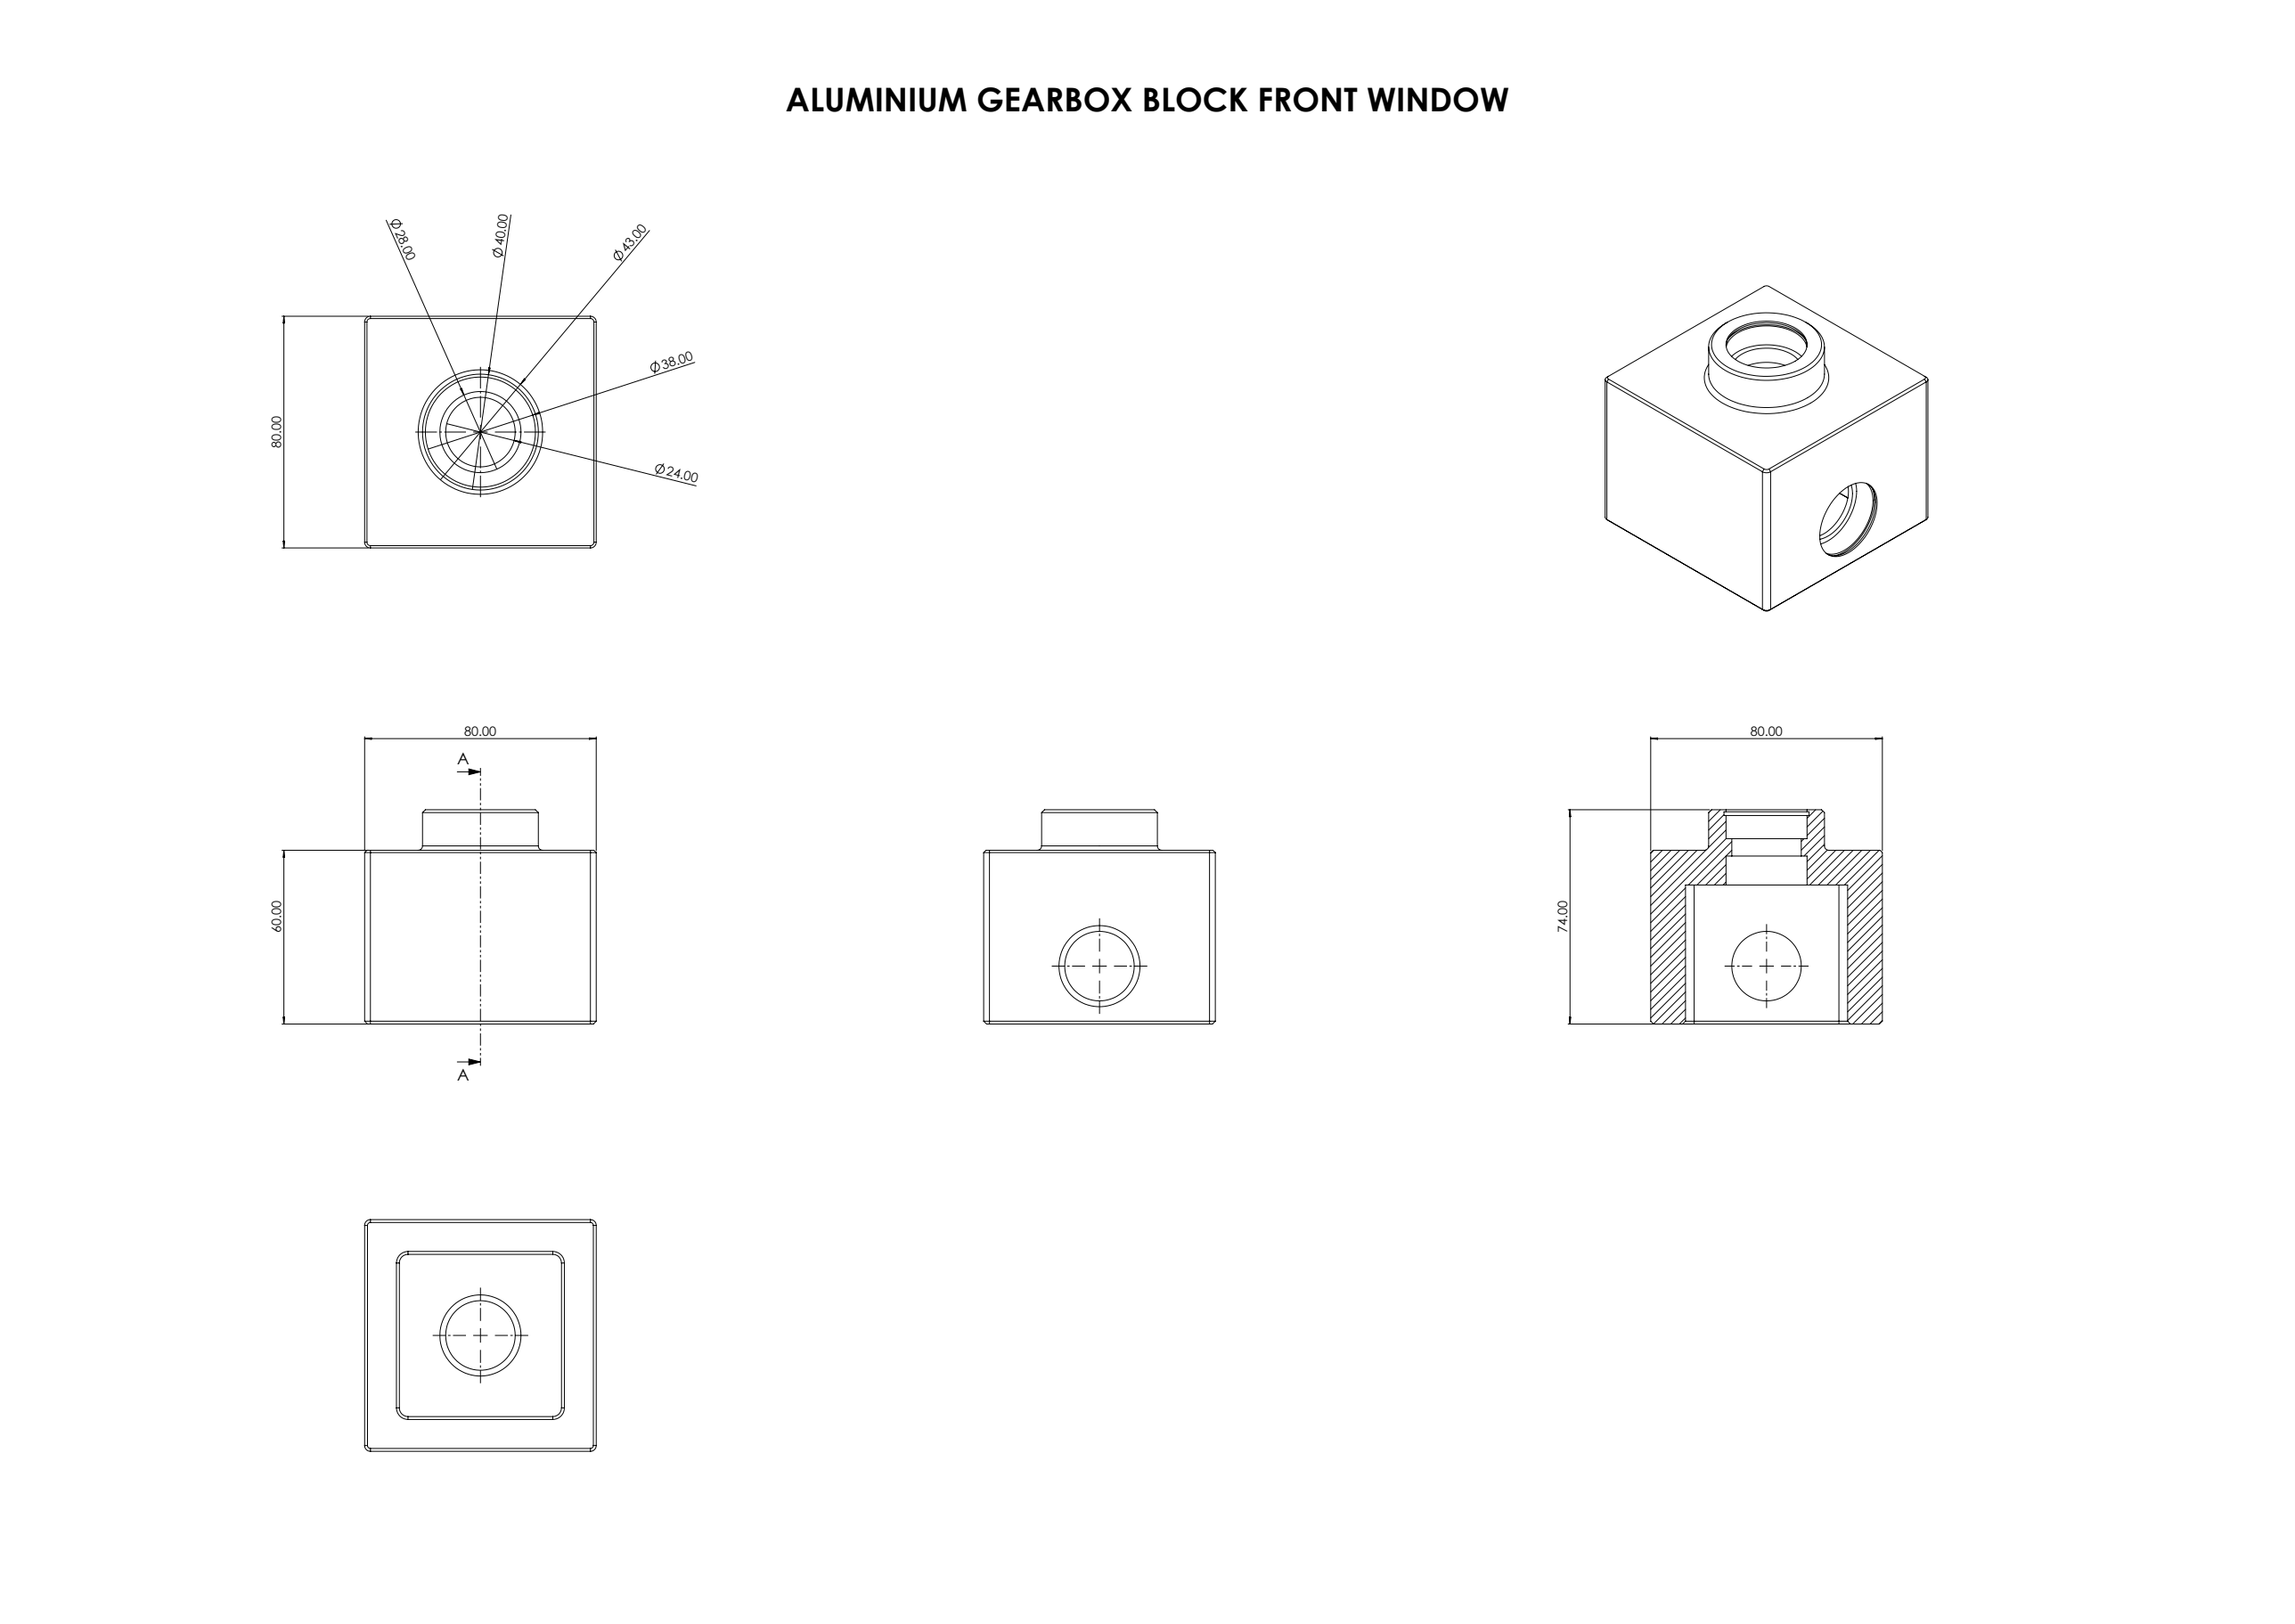
ISO-10303-21;
HEADER;
/* Generated by software containing ST-Developer
 * from STEP Tools, Inc. (www.steptools.com) 
 */

FILE_DESCRIPTION(
/* description */ (''),
/* implementation_level */ '2;1');

FILE_NAME(
/* name */ '01_Aluminium_Gearbox_Block_Front_Window.step',
/* time_stamp */ '2026-10-11T09:12:28-07:00',
/* author */ (''),
/* organization */ (''),
/* preprocessor_version */ 'ST-DEVELOPER v20.2',
/* originating_system */ 'Autodesk Translation Framework v15.15.0.0',
/* authorisation */ '');

FILE_SCHEMA (('AUTOMOTIVE_DESIGN { 1 0 10303 214 3 1 1 }'));
ENDSEC;

DATA;
#10=MECHANICAL_DESIGN_GEOMETRIC_PRESENTATION_REPRESENTATION('',(#647),#23254);
#627=SHAPE_REPRESENTATION_RELATIONSHIP('SRR','None',#23300,#637);
#637=ADVANCED_BREP_SHAPE_REPRESENTATION('',(#657),#23244);
#647=STYLED_ITEM('',(#23441),#657);
#657=MANIFOLD_SOLID_BREP('Body1',#7025);
#667=CONICAL_SURFACE('',#7210,19.5,0.785398163397451);
#668=CONICAL_SURFACE('',#7214,1.6,0.785398163397445);
#669=CONICAL_SURFACE('',#7217,1.6,0.785398163397448);
#670=CONICAL_SURFACE('',#7220,1.6,0.785398163397448);
#671=CONICAL_SURFACE('',#7223,1.6,0.785398163397445);
#672=CONICAL_SURFACE('',#7231,1.5,0.785398163397449);
#673=CONICAL_SURFACE('',#7234,1.5,0.785398163397447);
#674=CONICAL_SURFACE('',#7238,1.5,0.785398163397447);
#675=CONICAL_SURFACE('',#7242,1.5,0.785398163397449);
#676=CONICAL_SURFACE('',#7250,3.5,0.785398163397447);
#677=CONICAL_SURFACE('',#7253,3.5,0.785398163397447);
#678=CONICAL_SURFACE('',#7256,3.5,0.785398163397447);
#679=CONICAL_SURFACE('',#7259,3.5,0.785398163397447);
#759=TOROIDAL_SURFACE('',#7197,21.5,1.5);
#780=FACE_BOUND('',#1376,.T.);
#781=FACE_BOUND('',#1379,.T.);
#782=FACE_BOUND('',#1382,.T.);
#783=FACE_BOUND('',#1385,.T.);
#784=FACE_BOUND('',#1389,.T.);
#785=FACE_BOUND('',#1392,.T.);
#786=FACE_BOUND('',#1395,.T.);
#787=FACE_BOUND('',#1399,.T.);
#788=FACE_BOUND('',#1402,.T.);
#789=FACE_BOUND('',#1405,.T.);
#790=FACE_BOUND('',#1410,.T.);
#791=FACE_BOUND('',#1413,.T.);
#792=FACE_BOUND('',#1424,.T.);
#793=FACE_BOUND('',#1436,.T.);
#794=FACE_BOUND('',#1446,.T.);
#795=FACE_BOUND('',#1451,.T.);
#796=FACE_BOUND('',#1453,.T.);
#797=FACE_BOUND('',#1459,.T.);
#852=PLANE('',#7151);
#853=PLANE('',#7155);
#854=PLANE('',#7159);
#855=PLANE('',#7163);
#856=PLANE('',#7170);
#857=PLANE('',#7174);
#858=PLANE('',#7178);
#859=PLANE('',#7185);
#860=PLANE('',#7189);
#861=PLANE('',#7193);
#862=PLANE('',#7205);
#863=PLANE('',#7212);
#864=PLANE('',#7213);
#865=PLANE('',#7216);
#866=PLANE('',#7219);
#867=PLANE('',#7222);
#868=PLANE('',#7227);
#869=PLANE('',#7230);
#870=PLANE('',#7233);
#871=PLANE('',#7237);
#872=PLANE('',#7241);
#873=PLANE('',#7244);
#874=PLANE('',#7245);
#875=PLANE('',#7252);
#876=PLANE('',#7255);
#877=PLANE('',#7258);
#878=PLANE('',#7261);
#879=PLANE('',#7262);
#880=PLANE('',#7265);
#881=PLANE('',#7268);
#882=PLANE('',#7271);
#883=PLANE('',#7274);
#884=PLANE('',#7276);
#885=PLANE('',#7278);
#979=FACE_OUTER_BOUND('',#1374,.T.);
#980=FACE_OUTER_BOUND('',#1375,.T.);
#981=FACE_OUTER_BOUND('',#1377,.T.);
#982=FACE_OUTER_BOUND('',#1378,.T.);
#983=FACE_OUTER_BOUND('',#1380,.T.);
#984=FACE_OUTER_BOUND('',#1381,.T.);
#985=FACE_OUTER_BOUND('',#1383,.T.);
#986=FACE_OUTER_BOUND('',#1384,.T.);
#987=FACE_OUTER_BOUND('',#1386,.T.);
#988=FACE_OUTER_BOUND('',#1387,.T.);
#989=FACE_OUTER_BOUND('',#1388,.T.);
#990=FACE_OUTER_BOUND('',#1390,.T.);
#991=FACE_OUTER_BOUND('',#1391,.T.);
#992=FACE_OUTER_BOUND('',#1393,.T.);
#993=FACE_OUTER_BOUND('',#1394,.T.);
#994=FACE_OUTER_BOUND('',#1396,.T.);
#995=FACE_OUTER_BOUND('',#1397,.T.);
#996=FACE_OUTER_BOUND('',#1398,.T.);
#997=FACE_OUTER_BOUND('',#1400,.T.);
#998=FACE_OUTER_BOUND('',#1401,.T.);
#999=FACE_OUTER_BOUND('',#1403,.T.);
#1000=FACE_OUTER_BOUND('',#1404,.T.);
#1001=FACE_OUTER_BOUND('',#1406,.T.);
#1002=FACE_OUTER_BOUND('',#1407,.T.);
#1003=FACE_OUTER_BOUND('',#1408,.T.);
#1004=FACE_OUTER_BOUND('',#1409,.T.);
#1005=FACE_OUTER_BOUND('',#1411,.T.);
#1006=FACE_OUTER_BOUND('',#1412,.T.);
#1007=FACE_OUTER_BOUND('',#1414,.T.);
#1008=FACE_OUTER_BOUND('',#1415,.T.);
#1009=FACE_OUTER_BOUND('',#1416,.T.);
#1010=FACE_OUTER_BOUND('',#1417,.T.);
#1011=FACE_OUTER_BOUND('',#1418,.T.);
#1012=FACE_OUTER_BOUND('',#1419,.T.);
#1013=FACE_OUTER_BOUND('',#1420,.T.);
#1014=FACE_OUTER_BOUND('',#1421,.T.);
#1015=FACE_OUTER_BOUND('',#1422,.T.);
#1016=FACE_OUTER_BOUND('',#1423,.T.);
#1017=FACE_OUTER_BOUND('',#1425,.T.);
#1018=FACE_OUTER_BOUND('',#1426,.T.);
#1019=FACE_OUTER_BOUND('',#1427,.T.);
#1020=FACE_OUTER_BOUND('',#1428,.T.);
#1021=FACE_OUTER_BOUND('',#1429,.T.);
#1022=FACE_OUTER_BOUND('',#1430,.T.);
#1023=FACE_OUTER_BOUND('',#1431,.T.);
#1024=FACE_OUTER_BOUND('',#1432,.T.);
#1025=FACE_OUTER_BOUND('',#1433,.T.);
#1026=FACE_OUTER_BOUND('',#1434,.T.);
#1027=FACE_OUTER_BOUND('',#1435,.T.);
#1028=FACE_OUTER_BOUND('',#1437,.T.);
#1029=FACE_OUTER_BOUND('',#1438,.T.);
#1030=FACE_OUTER_BOUND('',#1439,.T.);
#1031=FACE_OUTER_BOUND('',#1440,.T.);
#1032=FACE_OUTER_BOUND('',#1441,.T.);
#1033=FACE_OUTER_BOUND('',#1442,.T.);
#1034=FACE_OUTER_BOUND('',#1443,.T.);
#1035=FACE_OUTER_BOUND('',#1444,.T.);
#1036=FACE_OUTER_BOUND('',#1445,.T.);
#1037=FACE_OUTER_BOUND('',#1447,.T.);
#1038=FACE_OUTER_BOUND('',#1448,.T.);
#1039=FACE_OUTER_BOUND('',#1449,.T.);
#1040=FACE_OUTER_BOUND('',#1450,.T.);
#1041=FACE_OUTER_BOUND('',#1452,.T.);
#1042=FACE_OUTER_BOUND('',#1454,.T.);
#1043=FACE_OUTER_BOUND('',#1455,.T.);
#1044=FACE_OUTER_BOUND('',#1456,.T.);
#1045=FACE_OUTER_BOUND('',#1457,.T.);
#1046=FACE_OUTER_BOUND('',#1458,.T.);
#1047=FACE_OUTER_BOUND('',#1460,.T.);
#1048=FACE_OUTER_BOUND('',#1461,.T.);
#1374=EDGE_LOOP('',(#4459,#4460,#4461,#4462));
#1375=EDGE_LOOP('',(#4463));
#1376=EDGE_LOOP('',(#4464));
#1377=EDGE_LOOP('',(#4465,#4466,#4467,#4468));
#1378=EDGE_LOOP('',(#4469));
#1379=EDGE_LOOP('',(#4470));
#1380=EDGE_LOOP('',(#4471,#4472,#4473,#4474));
#1381=EDGE_LOOP('',(#4475));
#1382=EDGE_LOOP('',(#4476));
#1383=EDGE_LOOP('',(#4477,#4478,#4479,#4480));
#1384=EDGE_LOOP('',(#4481));
#1385=EDGE_LOOP('',(#4482));
#1386=EDGE_LOOP('',(#4483,#4484,#4485,#4486));
#1387=EDGE_LOOP('',(#4487,#4488,#4489,#4490));
#1388=EDGE_LOOP('',(#4491));
#1389=EDGE_LOOP('',(#4492));
#1390=EDGE_LOOP('',(#4493,#4494,#4495,#4496));
#1391=EDGE_LOOP('',(#4497));
#1392=EDGE_LOOP('',(#4498));
#1393=EDGE_LOOP('',(#4499,#4500,#4501,#4502));
#1394=EDGE_LOOP('',(#4503));
#1395=EDGE_LOOP('',(#4504));
#1396=EDGE_LOOP('',(#4505,#4506,#4507,#4508));
#1397=EDGE_LOOP('',(#4509,#4510,#4511,#4512));
#1398=EDGE_LOOP('',(#4513));
#1399=EDGE_LOOP('',(#4514));
#1400=EDGE_LOOP('',(#4515,#4516,#4517,#4518));
#1401=EDGE_LOOP('',(#4519));
#1402=EDGE_LOOP('',(#4520));
#1403=EDGE_LOOP('',(#4521,#4522,#4523,#4524));
#1404=EDGE_LOOP('',(#4525));
#1405=EDGE_LOOP('',(#4526));
#1406=EDGE_LOOP('',(#4527,#4528,#4529,#4530));
#1407=EDGE_LOOP('',(#4531,#4532,#4533,#4534,#4535));
#1408=EDGE_LOOP('',(#4536,#4537,#4538,#4539,#4540,#4541));
#1409=EDGE_LOOP('',(#4542,#4543,#4544,#4545,#4546,#4547,#4548,#4549));
#1410=EDGE_LOOP('',(#4550));
#1411=EDGE_LOOP('',(#4551,#4552,#4553,#4554,#4555));
#1412=EDGE_LOOP('',(#4556));
#1413=EDGE_LOOP('',(#4557));
#1414=EDGE_LOOP('',(#4558,#4559,#4560,#4561));
#1415=EDGE_LOOP('',(#4562,#4563,#4564,#4565));
#1416=EDGE_LOOP('',(#4566,#4567,#4568,#4569));
#1417=EDGE_LOOP('',(#4570,#4571,#4572,#4573));
#1418=EDGE_LOOP('',(#4574,#4575,#4576,#4577));
#1419=EDGE_LOOP('',(#4578,#4579,#4580,#4581));
#1420=EDGE_LOOP('',(#4582,#4583,#4584,#4585));
#1421=EDGE_LOOP('',(#4586,#4587,#4588,#4589));
#1422=EDGE_LOOP('',(#4590,#4591,#4592,#4593));
#1423=EDGE_LOOP('',(#4594,#4595,#4596,#4597));
#1424=EDGE_LOOP('',(#4598));
#1425=EDGE_LOOP('',(#4599,#4600,#4601,#4602));
#1426=EDGE_LOOP('',(#4603,#4604,#4605,#4606));
#1427=EDGE_LOOP('',(#4607,#4608,#4609,#4610));
#1428=EDGE_LOOP('',(#4611,#4612,#4613,#4614));
#1429=EDGE_LOOP('',(#4615,#4616,#4617,#4618));
#1430=EDGE_LOOP('',(#4619,#4620,#4621,#4622));
#1431=EDGE_LOOP('',(#4623,#4624,#4625,#4626));
#1432=EDGE_LOOP('',(#4627,#4628,#4629,#4630));
#1433=EDGE_LOOP('',(#4631,#4632,#4633,#4634));
#1434=EDGE_LOOP('',(#4635,#4636,#4637,#4638));
#1435=EDGE_LOOP('',(#4639,#4640,#4641,#4642,#4643,#4644,#4645,#4646));
#1436=EDGE_LOOP('',(#4647,#4648,#4649,#4650,#4651,#4652,#4653,#4654));
#1437=EDGE_LOOP('',(#4655,#4656,#4657,#4658));
#1438=EDGE_LOOP('',(#4659,#4660,#4661,#4662));
#1439=EDGE_LOOP('',(#4663,#4664,#4665,#4666));
#1440=EDGE_LOOP('',(#4667,#4668,#4669,#4670));
#1441=EDGE_LOOP('',(#4671,#4672,#4673,#4674));
#1442=EDGE_LOOP('',(#4675,#4676,#4677,#4678));
#1443=EDGE_LOOP('',(#4679,#4680,#4681,#4682));
#1444=EDGE_LOOP('',(#4683,#4684,#4685,#4686));
#1445=EDGE_LOOP('',(#4687,#4688,#4689,#4690));
#1446=EDGE_LOOP('',(#4691));
#1447=EDGE_LOOP('',(#4692,#4693,#4694,#4695));
#1448=EDGE_LOOP('',(#4696,#4697,#4698,#4699));
#1449=EDGE_LOOP('',(#4700,#4701,#4702,#4703));
#1450=EDGE_LOOP('',(#4704,#4705,#4706,#4707,#4708,#4709,#4710,#4711));
#1451=EDGE_LOOP('',(#4712));
#1452=EDGE_LOOP('',(#4713,#4714,#4715,#4716));
#1453=EDGE_LOOP('',(#4717));
#1454=EDGE_LOOP('',(#4718,#4719,#4720,#4721));
#1455=EDGE_LOOP('',(#4722,#4723,#4724,#4725));
#1456=EDGE_LOOP('',(#4726,#4727,#4728,#4729));
#1457=EDGE_LOOP('',(#4730,#4731,#4732,#4733));
#1458=EDGE_LOOP('',(#4734,#4735,#4736,#4737));
#1459=EDGE_LOOP('',(#4738));
#1460=EDGE_LOOP('',(#4739,#4740,#4741,#4742));
#1461=EDGE_LOOP('',(#4743,#4744,#4745,#4746));
#1841=LINE('',#9466,#2100);
#1842=LINE('',#9473,#2101);
#1843=LINE('',#9480,#2102);
#1844=LINE('',#9487,#2103);
#1845=LINE('',#9494,#2104);
#1846=LINE('',#9500,#2105);
#1847=LINE('',#9507,#2106);
#1848=LINE('',#9514,#2107);
#1849=LINE('',#9521,#2108);
#1850=LINE('',#9527,#2109);
#1851=LINE('',#9534,#2110);
#1852=LINE('',#9541,#2111);
#1853=LINE('',#9548,#2112);
#1854=LINE('',#9560,#2113);
#1855=LINE('',#9567,#2114);
#1856=LINE('',#9571,#2115);
#1857=LINE('',#9575,#2116);
#1858=LINE('',#9579,#2117);
#1859=LINE('',#9583,#2118);
#1860=LINE('',#9588,#2119);
#1861=LINE('',#9590,#2120);
#1862=LINE('',#9591,#2121);
#1863=LINE('',#9595,#2122);
#1864=LINE('',#9598,#2123);
#1865=LINE('',#9599,#2124);
#1866=LINE('',#9603,#2125);
#1867=LINE('',#9606,#2126);
#1868=LINE('',#9607,#2127);
#1869=LINE('',#9611,#2128);
#1870=LINE('',#9614,#2129);
#1871=LINE('',#9615,#2130);
#1872=LINE('',#9620,#2131);
#1873=LINE('',#9623,#2132);
#1874=LINE('',#9626,#2133);
#1875=LINE('',#9627,#2134);
#1876=LINE('',#9630,#2135);
#1877=LINE('',#9634,#2136);
#1878=LINE('',#9635,#2137);
#1879=LINE('',#9638,#2138);
#1880=LINE('',#9640,#2139);
#1881=LINE('',#9645,#2140);
#1882=LINE('',#9646,#2141);
#1883=LINE('',#9647,#2142);
#1884=LINE('',#9651,#2143);
#1885=LINE('',#9656,#2144);
#1886=LINE('',#9658,#2145);
#1887=LINE('',#9659,#2146);
#1888=LINE('',#9662,#2147);
#1889=LINE('',#9667,#2148);
#1890=LINE('',#9668,#2149);
#1891=LINE('',#9671,#2150);
#1892=LINE('',#9674,#2151);
#1893=LINE('',#9680,#2152);
#1894=LINE('',#9684,#2153);
#1895=LINE('',#9688,#2154);
#1896=LINE('',#9691,#2155);
#1897=LINE('',#9694,#2156);
#1898=LINE('',#9697,#2157);
#1899=LINE('',#9700,#2158);
#1900=LINE('',#9701,#2159);
#1901=LINE('',#9704,#2160);
#1902=LINE('',#9708,#2161);
#1903=LINE('',#9709,#2162);
#1904=LINE('',#9712,#2163);
#1905=LINE('',#9716,#2164);
#1906=LINE('',#9717,#2165);
#1907=LINE('',#9720,#2166);
#1908=LINE('',#9723,#2167);
#1909=LINE('',#9726,#2168);
#1910=LINE('',#9728,#2169);
#1911=LINE('',#9729,#2170);
#1912=LINE('',#9732,#2171);
#1913=LINE('',#9736,#2172);
#1914=LINE('',#9737,#2173);
#1915=LINE('',#9740,#2174);
#1916=LINE('',#9744,#2175);
#1917=LINE('',#9748,#2176);
#1918=LINE('',#9751,#2177);
#1919=LINE('',#9753,#2178);
#1920=LINE('',#9755,#2179);
#1921=LINE('',#9758,#2180);
#1922=LINE('',#9759,#2181);
#1923=LINE('',#9761,#2182);
#2100=VECTOR('',#7839,14.);
#2101=VECTOR('',#7848,14.7);
#2102=VECTOR('',#7857,14.);
#2103=VECTOR('',#7866,12.);
#2104=VECTOR('',#7875,14.);
#2105=VECTOR('',#7882,14.);
#2106=VECTOR('',#7891,14.7);
#2107=VECTOR('',#7900,14.);
#2108=VECTOR('',#7909,12.);
#2109=VECTOR('',#7916,12.);
#2110=VECTOR('',#7925,14.);
#2111=VECTOR('',#7934,14.7);
#2112=VECTOR('',#7943,14.);
#2113=VECTOR('',#7958,20.);
#2114=VECTOR('',#7965,10.);
#2115=VECTOR('',#7968,10.);
#2116=VECTOR('',#7971,10.);
#2117=VECTOR('',#7974,10.);
#2118=VECTOR('',#7979,19.5);
#2119=VECTOR('',#7986,10.);
#2120=VECTOR('',#7987,10.);
#2121=VECTOR('',#7988,10.);
#2122=VECTOR('',#7993,10.);
#2123=VECTOR('',#7996,10.);
#2124=VECTOR('',#7997,10.);
#2125=VECTOR('',#8002,10.);
#2126=VECTOR('',#8005,10.);
#2127=VECTOR('',#8006,10.);
#2128=VECTOR('',#8011,10.);
#2129=VECTOR('',#8014,10.);
#2130=VECTOR('',#8015,10.);
#2131=VECTOR('',#8022,10.);
#2132=VECTOR('',#8025,10.);
#2133=VECTOR('',#8028,10.);
#2134=VECTOR('',#8029,10.);
#2135=VECTOR('',#8032,10.);
#2136=VECTOR('',#8037,10.);
#2137=VECTOR('',#8038,10.);
#2138=VECTOR('',#8041,10.);
#2139=VECTOR('',#8042,10.);
#2140=VECTOR('',#8047,10.);
#2141=VECTOR('',#8048,10.);
#2142=VECTOR('',#8049,10.);
#2143=VECTOR('',#8052,10.);
#2144=VECTOR('',#8059,10.);
#2145=VECTOR('',#8060,10.);
#2146=VECTOR('',#8061,10.);
#2147=VECTOR('',#8064,10.);
#2148=VECTOR('',#8071,10.);
#2149=VECTOR('',#8072,10.);
#2150=VECTOR('',#8075,10.);
#2151=VECTOR('',#8080,10.);
#2152=VECTOR('',#8085,10.);
#2153=VECTOR('',#8088,10.);
#2154=VECTOR('',#8091,10.);
#2155=VECTOR('',#8094,10.);
#2156=VECTOR('',#8097,10.);
#2157=VECTOR('',#8100,10.);
#2158=VECTOR('',#8103,10.);
#2159=VECTOR('',#8104,10.);
#2160=VECTOR('',#8107,10.);
#2161=VECTOR('',#8112,10.);
#2162=VECTOR('',#8113,10.);
#2163=VECTOR('',#8116,10.);
#2164=VECTOR('',#8121,10.);
#2165=VECTOR('',#8122,10.);
#2166=VECTOR('',#8125,10.);
#2167=VECTOR('',#8130,10.);
#2168=VECTOR('',#8133,10.);
#2169=VECTOR('',#8134,10.);
#2170=VECTOR('',#8135,10.);
#2171=VECTOR('',#8138,10.);
#2172=VECTOR('',#8143,10.);
#2173=VECTOR('',#8144,10.);
#2174=VECTOR('',#8147,10.);
#2175=VECTOR('',#8152,10.);
#2176=VECTOR('',#8155,10.);
#2177=VECTOR('',#8160,10.);
#2178=VECTOR('',#8163,10.);
#2179=VECTOR('',#8166,10.);
#2180=VECTOR('',#8171,10.);
#2181=VECTOR('',#8172,10.);
#2182=VECTOR('',#8175,10.);
#2359=CIRCLE('',#7149,14.);
#2360=CIRCLE('',#7150,14.);
#2361=CIRCLE('',#7152,14.7);
#2362=CIRCLE('',#7154,14.7);
#2363=CIRCLE('',#7156,14.);
#2364=CIRCLE('',#7158,14.);
#2365=CIRCLE('',#7160,12.);
#2366=CIRCLE('',#7162,12.);
#2367=CIRCLE('',#7164,14.);
#2368=CIRCLE('',#7166,14.);
#2369=CIRCLE('',#7168,14.);
#2370=CIRCLE('',#7169,14.);
#2371=CIRCLE('',#7171,14.7);
#2372=CIRCLE('',#7173,14.7);
#2373=CIRCLE('',#7175,14.);
#2374=CIRCLE('',#7177,14.);
#2375=CIRCLE('',#7179,12.);
#2376=CIRCLE('',#7181,12.);
#2377=CIRCLE('',#7183,12.);
#2378=CIRCLE('',#7184,12.);
#2379=CIRCLE('',#7186,14.);
#2380=CIRCLE('',#7188,14.);
#2381=CIRCLE('',#7190,14.7);
#2382=CIRCLE('',#7192,14.7);
#2383=CIRCLE('',#7194,14.);
#2384=CIRCLE('',#7196,14.);
#2385=CIRCLE('',#7198,20.);
#2386=CIRCLE('',#7199,1.5);
#2387=CIRCLE('',#7200,21.5);
#2388=CIRCLE('',#7201,20.);
#2389=CIRCLE('',#7203,20.);
#2390=CIRCLE('',#7204,20.);
#2391=CIRCLE('',#7206,1.2);
#2392=CIRCLE('',#7207,1.2);
#2393=CIRCLE('',#7208,1.2);
#2394=CIRCLE('',#7209,1.2);
#2395=CIRCLE('',#7211,19.);
#2396=CIRCLE('',#7215,2.);
#2397=CIRCLE('',#7218,2.);
#2398=CIRCLE('',#7221,2.);
#2399=CIRCLE('',#7224,2.);
#2400=CIRCLE('',#7226,2.);
#2401=CIRCLE('',#7229,2.);
#2402=CIRCLE('',#7232,1.);
#2403=CIRCLE('',#7235,2.);
#2404=CIRCLE('',#7236,1.);
#2405=CIRCLE('',#7239,2.);
#2406=CIRCLE('',#7240,1.);
#2407=CIRCLE('',#7243,1.);
#2408=CIRCLE('',#7246,4.);
#2409=CIRCLE('',#7247,4.);
#2410=CIRCLE('',#7248,4.);
#2411=CIRCLE('',#7249,4.);
#2412=CIRCLE('',#7251,3.);
#2413=CIRCLE('',#7254,3.);
#2414=CIRCLE('',#7257,3.);
#2415=CIRCLE('',#7260,3.);
#2416=CIRCLE('',#7264,3.);
#2417=CIRCLE('',#7267,3.);
#2418=CIRCLE('',#7269,3.);
#2419=CIRCLE('',#7270,3.);
#2702=VERTEX_POINT('',#9463);
#2703=VERTEX_POINT('',#9465);
#2704=VERTEX_POINT('',#9469);
#2705=VERTEX_POINT('',#9472);
#2706=VERTEX_POINT('',#9476);
#2707=VERTEX_POINT('',#9479);
#2708=VERTEX_POINT('',#9483);
#2709=VERTEX_POINT('',#9486);
#2710=VERTEX_POINT('',#9490);
#2711=VERTEX_POINT('',#9493);
#2712=VERTEX_POINT('',#9497);
#2713=VERTEX_POINT('',#9499);
#2714=VERTEX_POINT('',#9503);
#2715=VERTEX_POINT('',#9506);
#2716=VERTEX_POINT('',#9510);
#2717=VERTEX_POINT('',#9513);
#2718=VERTEX_POINT('',#9517);
#2719=VERTEX_POINT('',#9520);
#2720=VERTEX_POINT('',#9524);
#2721=VERTEX_POINT('',#9526);
#2722=VERTEX_POINT('',#9530);
#2723=VERTEX_POINT('',#9533);
#2724=VERTEX_POINT('',#9537);
#2725=VERTEX_POINT('',#9540);
#2726=VERTEX_POINT('',#9544);
#2727=VERTEX_POINT('',#9547);
#2728=VERTEX_POINT('',#9551);
#2729=VERTEX_POINT('',#9552);
#2730=VERTEX_POINT('',#9554);
#2731=VERTEX_POINT('',#9559);
#2732=VERTEX_POINT('',#9561);
#2733=VERTEX_POINT('',#9565);
#2734=VERTEX_POINT('',#9566);
#2735=VERTEX_POINT('',#9568);
#2736=VERTEX_POINT('',#9570);
#2737=VERTEX_POINT('',#9572);
#2738=VERTEX_POINT('',#9574);
#2739=VERTEX_POINT('',#9576);
#2740=VERTEX_POINT('',#9578);
#2741=VERTEX_POINT('',#9582);
#2742=VERTEX_POINT('',#9587);
#2743=VERTEX_POINT('',#9589);
#2744=VERTEX_POINT('',#9593);
#2745=VERTEX_POINT('',#9597);
#2746=VERTEX_POINT('',#9601);
#2747=VERTEX_POINT('',#9605);
#2748=VERTEX_POINT('',#9609);
#2749=VERTEX_POINT('',#9613);
#2750=VERTEX_POINT('',#9619);
#2751=VERTEX_POINT('',#9621);
#2752=VERTEX_POINT('',#9625);
#2753=VERTEX_POINT('',#9629);
#2754=VERTEX_POINT('',#9633);
#2755=VERTEX_POINT('',#9637);
#2756=VERTEX_POINT('',#9639);
#2757=VERTEX_POINT('',#9643);
#2758=VERTEX_POINT('',#9644);
#2759=VERTEX_POINT('',#9649);
#2760=VERTEX_POINT('',#9650);
#2761=VERTEX_POINT('',#9655);
#2762=VERTEX_POINT('',#9657);
#2763=VERTEX_POINT('',#9661);
#2764=VERTEX_POINT('',#9666);
#2765=VERTEX_POINT('',#9670);
#2766=VERTEX_POINT('',#9676);
#2767=VERTEX_POINT('',#9677);
#2768=VERTEX_POINT('',#9679);
#2769=VERTEX_POINT('',#9681);
#2770=VERTEX_POINT('',#9683);
#2771=VERTEX_POINT('',#9685);
#2772=VERTEX_POINT('',#9687);
#2773=VERTEX_POINT('',#9689);
#2774=VERTEX_POINT('',#9693);
#2775=VERTEX_POINT('',#9695);
#2776=VERTEX_POINT('',#9699);
#2777=VERTEX_POINT('',#9703);
#2778=VERTEX_POINT('',#9707);
#2779=VERTEX_POINT('',#9711);
#2780=VERTEX_POINT('',#9715);
#2781=VERTEX_POINT('',#9719);
#2782=VERTEX_POINT('',#9725);
#2783=VERTEX_POINT('',#9727);
#2784=VERTEX_POINT('',#9731);
#2785=VERTEX_POINT('',#9735);
#2786=VERTEX_POINT('',#9739);
#2787=VERTEX_POINT('',#9743);
#2788=VERTEX_POINT('',#9745);
#2789=VERTEX_POINT('',#9747);
#3405=EDGE_CURVE('',#2702,#2702,#2359,.T.);
#3406=EDGE_CURVE('',#2702,#2703,#1841,.T.);
#3407=EDGE_CURVE('',#2703,#2703,#2360,.T.);
#3408=EDGE_CURVE('',#2704,#2704,#2361,.T.);
#3409=EDGE_CURVE('',#2704,#2705,#1842,.T.);
#3410=EDGE_CURVE('',#2705,#2705,#2362,.T.);
#3411=EDGE_CURVE('',#2706,#2706,#2363,.T.);
#3412=EDGE_CURVE('',#2706,#2707,#1843,.T.);
#3413=EDGE_CURVE('',#2707,#2707,#2364,.T.);
#3414=EDGE_CURVE('',#2708,#2708,#2365,.T.);
#3415=EDGE_CURVE('',#2708,#2709,#1844,.T.);
#3416=EDGE_CURVE('',#2709,#2709,#2366,.T.);
#3417=EDGE_CURVE('',#2710,#2710,#2367,.T.);
#3418=EDGE_CURVE('',#2710,#2711,#1845,.T.);
#3419=EDGE_CURVE('',#2711,#2711,#2368,.T.);
#3420=EDGE_CURVE('',#2712,#2712,#2369,.T.);
#3421=EDGE_CURVE('',#2712,#2713,#1846,.T.);
#3422=EDGE_CURVE('',#2713,#2713,#2370,.T.);
#3423=EDGE_CURVE('',#2714,#2714,#2371,.T.);
#3424=EDGE_CURVE('',#2714,#2715,#1847,.T.);
#3425=EDGE_CURVE('',#2715,#2715,#2372,.T.);
#3426=EDGE_CURVE('',#2716,#2716,#2373,.T.);
#3427=EDGE_CURVE('',#2716,#2717,#1848,.T.);
#3428=EDGE_CURVE('',#2717,#2717,#2374,.T.);
#3429=EDGE_CURVE('',#2718,#2718,#2375,.T.);
#3430=EDGE_CURVE('',#2718,#2719,#1849,.T.);
#3431=EDGE_CURVE('',#2719,#2719,#2376,.T.);
#3432=EDGE_CURVE('',#2720,#2720,#2377,.T.);
#3433=EDGE_CURVE('',#2720,#2721,#1850,.T.);
#3434=EDGE_CURVE('',#2721,#2721,#2378,.T.);
#3435=EDGE_CURVE('',#2722,#2722,#2379,.T.);
#3436=EDGE_CURVE('',#2722,#2723,#1851,.T.);
#3437=EDGE_CURVE('',#2723,#2723,#2380,.T.);
#3438=EDGE_CURVE('',#2724,#2724,#2381,.T.);
#3439=EDGE_CURVE('',#2724,#2725,#1852,.T.);
#3440=EDGE_CURVE('',#2725,#2725,#2382,.T.);
#3441=EDGE_CURVE('',#2726,#2726,#2383,.T.);
#3442=EDGE_CURVE('',#2726,#2727,#1853,.T.);
#3443=EDGE_CURVE('',#2727,#2727,#2384,.T.);
#3444=EDGE_CURVE('',#2728,#2729,#2385,.T.);
#3445=EDGE_CURVE('',#2729,#2730,#2386,.T.);
#3446=EDGE_CURVE('',#2730,#2730,#2387,.T.);
#3447=EDGE_CURVE('',#2729,#2728,#2388,.T.);
#3448=EDGE_CURVE('',#2728,#2731,#1854,.T.);
#3449=EDGE_CURVE('',#2732,#2731,#2389,.T.);
#3450=EDGE_CURVE('',#2731,#2732,#2390,.T.);
#3451=EDGE_CURVE('',#2733,#2734,#1855,.T.);
#3452=EDGE_CURVE('',#2735,#2733,#2391,.T.);
#3453=EDGE_CURVE('',#2736,#2735,#1856,.T.);
#3454=EDGE_CURVE('',#2737,#2736,#2392,.T.);
#3455=EDGE_CURVE('',#2738,#2737,#1857,.T.);
#3456=EDGE_CURVE('',#2739,#2738,#2393,.T.);
#3457=EDGE_CURVE('',#2740,#2739,#1858,.T.);
#3458=EDGE_CURVE('',#2734,#2740,#2394,.T.);
#3459=EDGE_CURVE('',#2732,#2741,#1859,.T.);
#3460=EDGE_CURVE('',#2741,#2741,#2395,.T.);
#3461=EDGE_CURVE('',#2742,#2733,#1860,.T.);
#3462=EDGE_CURVE('',#2734,#2743,#1861,.T.);
#3463=EDGE_CURVE('',#2743,#2742,#1862,.T.);
#3464=EDGE_CURVE('',#2742,#2744,#2396,.T.);
#3465=EDGE_CURVE('',#2744,#2735,#1863,.T.);
#3466=EDGE_CURVE('',#2745,#2736,#1864,.T.);
#3467=EDGE_CURVE('',#2744,#2745,#1865,.T.);
#3468=EDGE_CURVE('',#2745,#2746,#2397,.T.);
#3469=EDGE_CURVE('',#2746,#2737,#1866,.T.);
#3470=EDGE_CURVE('',#2746,#2747,#1867,.T.);
#3471=EDGE_CURVE('',#2747,#2738,#1868,.T.);
#3472=EDGE_CURVE('',#2747,#2748,#2398,.T.);
#3473=EDGE_CURVE('',#2748,#2739,#1869,.T.);
#3474=EDGE_CURVE('',#2748,#2749,#1870,.T.);
#3475=EDGE_CURVE('',#2749,#2740,#1871,.T.);
#3476=EDGE_CURVE('',#2749,#2743,#2399,.T.);
#3477=EDGE_CURVE('',#2745,#2750,#1872,.T.);
#3478=EDGE_CURVE('',#2751,#2750,#2400,.T.);
#3479=EDGE_CURVE('',#2751,#2746,#1873,.T.);
#3480=EDGE_CURVE('',#2752,#2744,#1874,.T.);
#3481=EDGE_CURVE('',#2750,#2752,#1875,.T.);
#3482=EDGE_CURVE('',#2742,#2753,#1876,.T.);
#3483=EDGE_CURVE('',#2752,#2753,#2401,.T.);
#3484=EDGE_CURVE('',#2754,#2743,#1877,.T.);
#3485=EDGE_CURVE('',#2753,#2754,#1878,.T.);
#3486=EDGE_CURVE('',#2755,#2751,#1879,.T.);
#3487=EDGE_CURVE('',#2750,#2756,#1880,.T.);
#3488=EDGE_CURVE('',#2756,#2755,#2402,.T.);
#3489=EDGE_CURVE('',#2757,#2758,#1881,.T.);
#3490=EDGE_CURVE('',#2758,#2751,#1882,.T.);
#3491=EDGE_CURVE('',#2755,#2757,#1883,.T.);
#3492=EDGE_CURVE('',#2759,#2760,#1884,.T.);
#3493=EDGE_CURVE('',#2760,#2758,#2403,.T.);
#3494=EDGE_CURVE('',#2757,#2759,#2404,.T.);
#3495=EDGE_CURVE('',#2759,#2761,#1885,.T.);
#3496=EDGE_CURVE('',#2761,#2762,#1886,.T.);
#3497=EDGE_CURVE('',#2762,#2760,#1887,.T.);
#3498=EDGE_CURVE('',#2763,#2754,#1888,.T.);
#3499=EDGE_CURVE('',#2754,#2762,#2405,.T.);
#3500=EDGE_CURVE('',#2761,#2763,#2406,.T.);
#3501=EDGE_CURVE('',#2763,#2764,#1889,.T.);
#3502=EDGE_CURVE('',#2764,#2753,#1890,.T.);
#3503=EDGE_CURVE('',#2765,#2752,#1891,.T.);
#3504=EDGE_CURVE('',#2764,#2765,#2407,.T.);
#3505=EDGE_CURVE('',#2765,#2756,#1892,.T.);
#3506=EDGE_CURVE('',#2766,#2767,#2408,.T.);
#3507=EDGE_CURVE('',#2768,#2766,#1893,.T.);
#3508=EDGE_CURVE('',#2769,#2768,#2409,.T.);
#3509=EDGE_CURVE('',#2770,#2769,#1894,.T.);
#3510=EDGE_CURVE('',#2771,#2770,#2410,.T.);
#3511=EDGE_CURVE('',#2772,#2771,#1895,.T.);
#3512=EDGE_CURVE('',#2773,#2772,#2411,.T.);
#3513=EDGE_CURVE('',#2767,#2773,#1896,.T.);
#3514=EDGE_CURVE('',#2767,#2774,#1897,.T.);
#3515=EDGE_CURVE('',#2774,#2775,#2412,.T.);
#3516=EDGE_CURVE('',#2775,#2766,#1898,.T.);
#3517=EDGE_CURVE('',#2773,#2776,#1899,.T.);
#3518=EDGE_CURVE('',#2776,#2774,#1900,.T.);
#3519=EDGE_CURVE('',#2772,#2777,#1901,.T.);
#3520=EDGE_CURVE('',#2777,#2776,#2413,.T.);
#3521=EDGE_CURVE('',#2771,#2778,#1902,.T.);
#3522=EDGE_CURVE('',#2778,#2777,#1903,.T.);
#3523=EDGE_CURVE('',#2770,#2779,#1904,.T.);
#3524=EDGE_CURVE('',#2779,#2778,#2414,.T.);
#3525=EDGE_CURVE('',#2769,#2780,#1905,.T.);
#3526=EDGE_CURVE('',#2780,#2779,#1906,.T.);
#3527=EDGE_CURVE('',#2768,#2781,#1907,.T.);
#3528=EDGE_CURVE('',#2781,#2780,#2415,.T.);
#3529=EDGE_CURVE('',#2775,#2781,#1908,.T.);
#3530=EDGE_CURVE('',#2782,#2780,#1909,.T.);
#3531=EDGE_CURVE('',#2783,#2782,#1910,.T.);
#3532=EDGE_CURVE('',#2779,#2783,#1911,.T.);
#3533=EDGE_CURVE('',#2781,#2784,#1912,.T.);
#3534=EDGE_CURVE('',#2782,#2784,#2416,.T.);
#3535=EDGE_CURVE('',#2785,#2775,#1913,.T.);
#3536=EDGE_CURVE('',#2784,#2785,#1914,.T.);
#3537=EDGE_CURVE('',#2774,#2786,#1915,.T.);
#3538=EDGE_CURVE('',#2785,#2786,#2417,.T.);
#3539=EDGE_CURVE('',#2787,#2786,#1916,.T.);
#3540=EDGE_CURVE('',#2787,#2788,#2418,.T.);
#3541=EDGE_CURVE('',#2789,#2788,#1917,.T.);
#3542=EDGE_CURVE('',#2789,#2783,#2419,.T.);
#3543=EDGE_CURVE('',#2787,#2776,#1918,.T.);
#3544=EDGE_CURVE('',#2777,#2788,#1919,.T.);
#3545=EDGE_CURVE('',#2789,#2778,#1920,.T.);
#3546=EDGE_CURVE('',#2747,#2758,#1921,.T.);
#3547=EDGE_CURVE('',#2760,#2748,#1922,.T.);
#3548=EDGE_CURVE('',#2749,#2762,#1923,.T.);
#4459=ORIENTED_EDGE('',*,*,#3405,.F.);
#4460=ORIENTED_EDGE('',*,*,#3406,.T.);
#4461=ORIENTED_EDGE('',*,*,#3407,.T.);
#4462=ORIENTED_EDGE('',*,*,#3406,.F.);
#4463=ORIENTED_EDGE('',*,*,#3408,.T.);
#4464=ORIENTED_EDGE('',*,*,#3407,.F.);
#4465=ORIENTED_EDGE('',*,*,#3408,.F.);
#4466=ORIENTED_EDGE('',*,*,#3409,.T.);
#4467=ORIENTED_EDGE('',*,*,#3410,.T.);
#4468=ORIENTED_EDGE('',*,*,#3409,.F.);
#4469=ORIENTED_EDGE('',*,*,#3410,.F.);
#4470=ORIENTED_EDGE('',*,*,#3411,.T.);
#4471=ORIENTED_EDGE('',*,*,#3411,.F.);
#4472=ORIENTED_EDGE('',*,*,#3412,.T.);
#4473=ORIENTED_EDGE('',*,*,#3413,.T.);
#4474=ORIENTED_EDGE('',*,*,#3412,.F.);
#4475=ORIENTED_EDGE('',*,*,#3413,.F.);
#4476=ORIENTED_EDGE('',*,*,#3414,.T.);
#4477=ORIENTED_EDGE('',*,*,#3414,.F.);
#4478=ORIENTED_EDGE('',*,*,#3415,.T.);
#4479=ORIENTED_EDGE('',*,*,#3416,.T.);
#4480=ORIENTED_EDGE('',*,*,#3415,.F.);
#4481=ORIENTED_EDGE('',*,*,#3417,.T.);
#4482=ORIENTED_EDGE('',*,*,#3416,.F.);
#4483=ORIENTED_EDGE('',*,*,#3417,.F.);
#4484=ORIENTED_EDGE('',*,*,#3418,.T.);
#4485=ORIENTED_EDGE('',*,*,#3419,.F.);
#4486=ORIENTED_EDGE('',*,*,#3418,.F.);
#4487=ORIENTED_EDGE('',*,*,#3420,.F.);
#4488=ORIENTED_EDGE('',*,*,#3421,.T.);
#4489=ORIENTED_EDGE('',*,*,#3422,.T.);
#4490=ORIENTED_EDGE('',*,*,#3421,.F.);
#4491=ORIENTED_EDGE('',*,*,#3423,.T.);
#4492=ORIENTED_EDGE('',*,*,#3422,.F.);
#4493=ORIENTED_EDGE('',*,*,#3423,.F.);
#4494=ORIENTED_EDGE('',*,*,#3424,.T.);
#4495=ORIENTED_EDGE('',*,*,#3425,.T.);
#4496=ORIENTED_EDGE('',*,*,#3424,.F.);
#4497=ORIENTED_EDGE('',*,*,#3425,.F.);
#4498=ORIENTED_EDGE('',*,*,#3426,.T.);
#4499=ORIENTED_EDGE('',*,*,#3426,.F.);
#4500=ORIENTED_EDGE('',*,*,#3427,.T.);
#4501=ORIENTED_EDGE('',*,*,#3428,.T.);
#4502=ORIENTED_EDGE('',*,*,#3427,.F.);
#4503=ORIENTED_EDGE('',*,*,#3428,.F.);
#4504=ORIENTED_EDGE('',*,*,#3429,.T.);
#4505=ORIENTED_EDGE('',*,*,#3429,.F.);
#4506=ORIENTED_EDGE('',*,*,#3430,.T.);
#4507=ORIENTED_EDGE('',*,*,#3431,.F.);
#4508=ORIENTED_EDGE('',*,*,#3430,.F.);
#4509=ORIENTED_EDGE('',*,*,#3432,.F.);
#4510=ORIENTED_EDGE('',*,*,#3433,.T.);
#4511=ORIENTED_EDGE('',*,*,#3434,.T.);
#4512=ORIENTED_EDGE('',*,*,#3433,.F.);
#4513=ORIENTED_EDGE('',*,*,#3435,.T.);
#4514=ORIENTED_EDGE('',*,*,#3434,.F.);
#4515=ORIENTED_EDGE('',*,*,#3435,.F.);
#4516=ORIENTED_EDGE('',*,*,#3436,.T.);
#4517=ORIENTED_EDGE('',*,*,#3437,.T.);
#4518=ORIENTED_EDGE('',*,*,#3436,.F.);
#4519=ORIENTED_EDGE('',*,*,#3438,.T.);
#4520=ORIENTED_EDGE('',*,*,#3437,.F.);
#4521=ORIENTED_EDGE('',*,*,#3438,.F.);
#4522=ORIENTED_EDGE('',*,*,#3439,.T.);
#4523=ORIENTED_EDGE('',*,*,#3440,.T.);
#4524=ORIENTED_EDGE('',*,*,#3439,.F.);
#4525=ORIENTED_EDGE('',*,*,#3440,.F.);
#4526=ORIENTED_EDGE('',*,*,#3441,.T.);
#4527=ORIENTED_EDGE('',*,*,#3441,.F.);
#4528=ORIENTED_EDGE('',*,*,#3442,.T.);
#4529=ORIENTED_EDGE('',*,*,#3443,.F.);
#4530=ORIENTED_EDGE('',*,*,#3442,.F.);
#4531=ORIENTED_EDGE('',*,*,#3444,.T.);
#4532=ORIENTED_EDGE('',*,*,#3445,.T.);
#4533=ORIENTED_EDGE('',*,*,#3446,.T.);
#4534=ORIENTED_EDGE('',*,*,#3445,.F.);
#4535=ORIENTED_EDGE('',*,*,#3447,.T.);
#4536=ORIENTED_EDGE('',*,*,#3444,.F.);
#4537=ORIENTED_EDGE('',*,*,#3448,.T.);
#4538=ORIENTED_EDGE('',*,*,#3449,.F.);
#4539=ORIENTED_EDGE('',*,*,#3450,.F.);
#4540=ORIENTED_EDGE('',*,*,#3448,.F.);
#4541=ORIENTED_EDGE('',*,*,#3447,.F.);
#4542=ORIENTED_EDGE('',*,*,#3451,.F.);
#4543=ORIENTED_EDGE('',*,*,#3452,.F.);
#4544=ORIENTED_EDGE('',*,*,#3453,.F.);
#4545=ORIENTED_EDGE('',*,*,#3454,.F.);
#4546=ORIENTED_EDGE('',*,*,#3455,.F.);
#4547=ORIENTED_EDGE('',*,*,#3456,.F.);
#4548=ORIENTED_EDGE('',*,*,#3457,.F.);
#4549=ORIENTED_EDGE('',*,*,#3458,.F.);
#4550=ORIENTED_EDGE('',*,*,#3446,.F.);
#4551=ORIENTED_EDGE('',*,*,#3449,.T.);
#4552=ORIENTED_EDGE('',*,*,#3450,.T.);
#4553=ORIENTED_EDGE('',*,*,#3459,.T.);
#4554=ORIENTED_EDGE('',*,*,#3460,.T.);
#4555=ORIENTED_EDGE('',*,*,#3459,.F.);
#4556=ORIENTED_EDGE('',*,*,#3460,.F.);
#4557=ORIENTED_EDGE('',*,*,#3405,.T.);
#4558=ORIENTED_EDGE('',*,*,#3461,.T.);
#4559=ORIENTED_EDGE('',*,*,#3451,.T.);
#4560=ORIENTED_EDGE('',*,*,#3462,.T.);
#4561=ORIENTED_EDGE('',*,*,#3463,.T.);
#4562=ORIENTED_EDGE('',*,*,#3461,.F.);
#4563=ORIENTED_EDGE('',*,*,#3464,.T.);
#4564=ORIENTED_EDGE('',*,*,#3465,.T.);
#4565=ORIENTED_EDGE('',*,*,#3452,.T.);
#4566=ORIENTED_EDGE('',*,*,#3466,.T.);
#4567=ORIENTED_EDGE('',*,*,#3453,.T.);
#4568=ORIENTED_EDGE('',*,*,#3465,.F.);
#4569=ORIENTED_EDGE('',*,*,#3467,.T.);
#4570=ORIENTED_EDGE('',*,*,#3466,.F.);
#4571=ORIENTED_EDGE('',*,*,#3468,.T.);
#4572=ORIENTED_EDGE('',*,*,#3469,.T.);
#4573=ORIENTED_EDGE('',*,*,#3454,.T.);
#4574=ORIENTED_EDGE('',*,*,#3469,.F.);
#4575=ORIENTED_EDGE('',*,*,#3470,.T.);
#4576=ORIENTED_EDGE('',*,*,#3471,.T.);
#4577=ORIENTED_EDGE('',*,*,#3455,.T.);
#4578=ORIENTED_EDGE('',*,*,#3471,.F.);
#4579=ORIENTED_EDGE('',*,*,#3472,.T.);
#4580=ORIENTED_EDGE('',*,*,#3473,.T.);
#4581=ORIENTED_EDGE('',*,*,#3456,.T.);
#4582=ORIENTED_EDGE('',*,*,#3473,.F.);
#4583=ORIENTED_EDGE('',*,*,#3474,.T.);
#4584=ORIENTED_EDGE('',*,*,#3475,.T.);
#4585=ORIENTED_EDGE('',*,*,#3457,.T.);
#4586=ORIENTED_EDGE('',*,*,#3475,.F.);
#4587=ORIENTED_EDGE('',*,*,#3476,.T.);
#4588=ORIENTED_EDGE('',*,*,#3462,.F.);
#4589=ORIENTED_EDGE('',*,*,#3458,.T.);
#4590=ORIENTED_EDGE('',*,*,#3468,.F.);
#4591=ORIENTED_EDGE('',*,*,#3477,.T.);
#4592=ORIENTED_EDGE('',*,*,#3478,.F.);
#4593=ORIENTED_EDGE('',*,*,#3479,.T.);
#4594=ORIENTED_EDGE('',*,*,#3467,.F.);
#4595=ORIENTED_EDGE('',*,*,#3480,.F.);
#4596=ORIENTED_EDGE('',*,*,#3481,.F.);
#4597=ORIENTED_EDGE('',*,*,#3477,.F.);
#4598=ORIENTED_EDGE('',*,*,#3420,.T.);
#4599=ORIENTED_EDGE('',*,*,#3464,.F.);
#4600=ORIENTED_EDGE('',*,*,#3482,.T.);
#4601=ORIENTED_EDGE('',*,*,#3483,.F.);
#4602=ORIENTED_EDGE('',*,*,#3480,.T.);
#4603=ORIENTED_EDGE('',*,*,#3463,.F.);
#4604=ORIENTED_EDGE('',*,*,#3484,.F.);
#4605=ORIENTED_EDGE('',*,*,#3485,.F.);
#4606=ORIENTED_EDGE('',*,*,#3482,.F.);
#4607=ORIENTED_EDGE('',*,*,#3486,.T.);
#4608=ORIENTED_EDGE('',*,*,#3478,.T.);
#4609=ORIENTED_EDGE('',*,*,#3487,.T.);
#4610=ORIENTED_EDGE('',*,*,#3488,.T.);
#4611=ORIENTED_EDGE('',*,*,#3489,.T.);
#4612=ORIENTED_EDGE('',*,*,#3490,.T.);
#4613=ORIENTED_EDGE('',*,*,#3486,.F.);
#4614=ORIENTED_EDGE('',*,*,#3491,.T.);
#4615=ORIENTED_EDGE('',*,*,#3492,.T.);
#4616=ORIENTED_EDGE('',*,*,#3493,.T.);
#4617=ORIENTED_EDGE('',*,*,#3489,.F.);
#4618=ORIENTED_EDGE('',*,*,#3494,.T.);
#4619=ORIENTED_EDGE('',*,*,#3492,.F.);
#4620=ORIENTED_EDGE('',*,*,#3495,.T.);
#4621=ORIENTED_EDGE('',*,*,#3496,.T.);
#4622=ORIENTED_EDGE('',*,*,#3497,.T.);
#4623=ORIENTED_EDGE('',*,*,#3498,.T.);
#4624=ORIENTED_EDGE('',*,*,#3499,.T.);
#4625=ORIENTED_EDGE('',*,*,#3496,.F.);
#4626=ORIENTED_EDGE('',*,*,#3500,.T.);
#4627=ORIENTED_EDGE('',*,*,#3498,.F.);
#4628=ORIENTED_EDGE('',*,*,#3501,.T.);
#4629=ORIENTED_EDGE('',*,*,#3502,.T.);
#4630=ORIENTED_EDGE('',*,*,#3485,.T.);
#4631=ORIENTED_EDGE('',*,*,#3503,.T.);
#4632=ORIENTED_EDGE('',*,*,#3483,.T.);
#4633=ORIENTED_EDGE('',*,*,#3502,.F.);
#4634=ORIENTED_EDGE('',*,*,#3504,.T.);
#4635=ORIENTED_EDGE('',*,*,#3487,.F.);
#4636=ORIENTED_EDGE('',*,*,#3481,.T.);
#4637=ORIENTED_EDGE('',*,*,#3503,.F.);
#4638=ORIENTED_EDGE('',*,*,#3505,.T.);
#4639=ORIENTED_EDGE('',*,*,#3488,.F.);
#4640=ORIENTED_EDGE('',*,*,#3505,.F.);
#4641=ORIENTED_EDGE('',*,*,#3504,.F.);
#4642=ORIENTED_EDGE('',*,*,#3501,.F.);
#4643=ORIENTED_EDGE('',*,*,#3500,.F.);
#4644=ORIENTED_EDGE('',*,*,#3495,.F.);
#4645=ORIENTED_EDGE('',*,*,#3494,.F.);
#4646=ORIENTED_EDGE('',*,*,#3491,.F.);
#4647=ORIENTED_EDGE('',*,*,#3506,.F.);
#4648=ORIENTED_EDGE('',*,*,#3507,.F.);
#4649=ORIENTED_EDGE('',*,*,#3508,.F.);
#4650=ORIENTED_EDGE('',*,*,#3509,.F.);
#4651=ORIENTED_EDGE('',*,*,#3510,.F.);
#4652=ORIENTED_EDGE('',*,*,#3511,.F.);
#4653=ORIENTED_EDGE('',*,*,#3512,.F.);
#4654=ORIENTED_EDGE('',*,*,#3513,.F.);
#4655=ORIENTED_EDGE('',*,*,#3514,.T.);
#4656=ORIENTED_EDGE('',*,*,#3515,.T.);
#4657=ORIENTED_EDGE('',*,*,#3516,.T.);
#4658=ORIENTED_EDGE('',*,*,#3506,.T.);
#4659=ORIENTED_EDGE('',*,*,#3514,.F.);
#4660=ORIENTED_EDGE('',*,*,#3513,.T.);
#4661=ORIENTED_EDGE('',*,*,#3517,.T.);
#4662=ORIENTED_EDGE('',*,*,#3518,.T.);
#4663=ORIENTED_EDGE('',*,*,#3519,.T.);
#4664=ORIENTED_EDGE('',*,*,#3520,.T.);
#4665=ORIENTED_EDGE('',*,*,#3517,.F.);
#4666=ORIENTED_EDGE('',*,*,#3512,.T.);
#4667=ORIENTED_EDGE('',*,*,#3519,.F.);
#4668=ORIENTED_EDGE('',*,*,#3511,.T.);
#4669=ORIENTED_EDGE('',*,*,#3521,.T.);
#4670=ORIENTED_EDGE('',*,*,#3522,.T.);
#4671=ORIENTED_EDGE('',*,*,#3523,.T.);
#4672=ORIENTED_EDGE('',*,*,#3524,.T.);
#4673=ORIENTED_EDGE('',*,*,#3521,.F.);
#4674=ORIENTED_EDGE('',*,*,#3510,.T.);
#4675=ORIENTED_EDGE('',*,*,#3523,.F.);
#4676=ORIENTED_EDGE('',*,*,#3509,.T.);
#4677=ORIENTED_EDGE('',*,*,#3525,.T.);
#4678=ORIENTED_EDGE('',*,*,#3526,.T.);
#4679=ORIENTED_EDGE('',*,*,#3527,.T.);
#4680=ORIENTED_EDGE('',*,*,#3528,.T.);
#4681=ORIENTED_EDGE('',*,*,#3525,.F.);
#4682=ORIENTED_EDGE('',*,*,#3508,.T.);
#4683=ORIENTED_EDGE('',*,*,#3527,.F.);
#4684=ORIENTED_EDGE('',*,*,#3507,.T.);
#4685=ORIENTED_EDGE('',*,*,#3516,.F.);
#4686=ORIENTED_EDGE('',*,*,#3529,.T.);
#4687=ORIENTED_EDGE('',*,*,#3526,.F.);
#4688=ORIENTED_EDGE('',*,*,#3530,.F.);
#4689=ORIENTED_EDGE('',*,*,#3531,.F.);
#4690=ORIENTED_EDGE('',*,*,#3532,.F.);
#4691=ORIENTED_EDGE('',*,*,#3432,.T.);
#4692=ORIENTED_EDGE('',*,*,#3528,.F.);
#4693=ORIENTED_EDGE('',*,*,#3533,.T.);
#4694=ORIENTED_EDGE('',*,*,#3534,.F.);
#4695=ORIENTED_EDGE('',*,*,#3530,.T.);
#4696=ORIENTED_EDGE('',*,*,#3529,.F.);
#4697=ORIENTED_EDGE('',*,*,#3535,.F.);
#4698=ORIENTED_EDGE('',*,*,#3536,.F.);
#4699=ORIENTED_EDGE('',*,*,#3533,.F.);
#4700=ORIENTED_EDGE('',*,*,#3515,.F.);
#4701=ORIENTED_EDGE('',*,*,#3537,.T.);
#4702=ORIENTED_EDGE('',*,*,#3538,.F.);
#4703=ORIENTED_EDGE('',*,*,#3535,.T.);
#4704=ORIENTED_EDGE('',*,*,#3538,.T.);
#4705=ORIENTED_EDGE('',*,*,#3539,.F.);
#4706=ORIENTED_EDGE('',*,*,#3540,.T.);
#4707=ORIENTED_EDGE('',*,*,#3541,.F.);
#4708=ORIENTED_EDGE('',*,*,#3542,.T.);
#4709=ORIENTED_EDGE('',*,*,#3531,.T.);
#4710=ORIENTED_EDGE('',*,*,#3534,.T.);
#4711=ORIENTED_EDGE('',*,*,#3536,.T.);
#4712=ORIENTED_EDGE('',*,*,#3419,.T.);
#4713=ORIENTED_EDGE('',*,*,#3518,.F.);
#4714=ORIENTED_EDGE('',*,*,#3543,.F.);
#4715=ORIENTED_EDGE('',*,*,#3539,.T.);
#4716=ORIENTED_EDGE('',*,*,#3537,.F.);
#4717=ORIENTED_EDGE('',*,*,#3431,.T.);
#4718=ORIENTED_EDGE('',*,*,#3520,.F.);
#4719=ORIENTED_EDGE('',*,*,#3544,.T.);
#4720=ORIENTED_EDGE('',*,*,#3540,.F.);
#4721=ORIENTED_EDGE('',*,*,#3543,.T.);
#4722=ORIENTED_EDGE('',*,*,#3524,.F.);
#4723=ORIENTED_EDGE('',*,*,#3532,.T.);
#4724=ORIENTED_EDGE('',*,*,#3542,.F.);
#4725=ORIENTED_EDGE('',*,*,#3545,.T.);
#4726=ORIENTED_EDGE('',*,*,#3522,.F.);
#4727=ORIENTED_EDGE('',*,*,#3545,.F.);
#4728=ORIENTED_EDGE('',*,*,#3541,.T.);
#4729=ORIENTED_EDGE('',*,*,#3544,.F.);
#4730=ORIENTED_EDGE('',*,*,#3472,.F.);
#4731=ORIENTED_EDGE('',*,*,#3546,.T.);
#4732=ORIENTED_EDGE('',*,*,#3493,.F.);
#4733=ORIENTED_EDGE('',*,*,#3547,.T.);
#4734=ORIENTED_EDGE('',*,*,#3474,.F.);
#4735=ORIENTED_EDGE('',*,*,#3547,.F.);
#4736=ORIENTED_EDGE('',*,*,#3497,.F.);
#4737=ORIENTED_EDGE('',*,*,#3548,.F.);
#4738=ORIENTED_EDGE('',*,*,#3443,.T.);
#4739=ORIENTED_EDGE('',*,*,#3476,.F.);
#4740=ORIENTED_EDGE('',*,*,#3548,.T.);
#4741=ORIENTED_EDGE('',*,*,#3499,.F.);
#4742=ORIENTED_EDGE('',*,*,#3484,.T.);
#4743=ORIENTED_EDGE('',*,*,#3470,.F.);
#4744=ORIENTED_EDGE('',*,*,#3479,.F.);
#4745=ORIENTED_EDGE('',*,*,#3490,.F.);
#4746=ORIENTED_EDGE('',*,*,#3546,.F.);
#6567=CYLINDRICAL_SURFACE('',#7148,14.);
#6568=CYLINDRICAL_SURFACE('',#7153,14.7);
#6569=CYLINDRICAL_SURFACE('',#7157,14.);
#6570=CYLINDRICAL_SURFACE('',#7161,12.);
#6571=CYLINDRICAL_SURFACE('',#7165,14.);
#6572=CYLINDRICAL_SURFACE('',#7167,14.);
#6573=CYLINDRICAL_SURFACE('',#7172,14.7);
#6574=CYLINDRICAL_SURFACE('',#7176,14.);
#6575=CYLINDRICAL_SURFACE('',#7180,12.);
#6576=CYLINDRICAL_SURFACE('',#7182,12.);
#6577=CYLINDRICAL_SURFACE('',#7187,14.);
#6578=CYLINDRICAL_SURFACE('',#7191,14.7);
#6579=CYLINDRICAL_SURFACE('',#7195,14.);
#6580=CYLINDRICAL_SURFACE('',#7202,20.);
#6581=CYLINDRICAL_SURFACE('',#7225,2.);
#6582=CYLINDRICAL_SURFACE('',#7228,2.);
#6583=CYLINDRICAL_SURFACE('',#7263,3.);
#6584=CYLINDRICAL_SURFACE('',#7266,3.);
#6585=CYLINDRICAL_SURFACE('',#7272,3.);
#6586=CYLINDRICAL_SURFACE('',#7273,3.);
#6587=CYLINDRICAL_SURFACE('',#7275,2.);
#6588=CYLINDRICAL_SURFACE('',#7277,2.);
#6630=ADVANCED_FACE('',(#979),#6567,.F.);
#6631=ADVANCED_FACE('',(#980,#780),#852,.F.);
#6632=ADVANCED_FACE('',(#981),#6568,.F.);
#6633=ADVANCED_FACE('',(#982,#781),#853,.F.);
#6634=ADVANCED_FACE('',(#983),#6569,.F.);
#6635=ADVANCED_FACE('',(#984,#782),#854,.F.);
#6636=ADVANCED_FACE('',(#985),#6570,.F.);
#6637=ADVANCED_FACE('',(#986,#783),#855,.F.);
#6638=ADVANCED_FACE('',(#987),#6571,.F.);
#6639=ADVANCED_FACE('',(#988),#6572,.F.);
#6640=ADVANCED_FACE('',(#989,#784),#856,.F.);
#6641=ADVANCED_FACE('',(#990),#6573,.F.);
#6642=ADVANCED_FACE('',(#991,#785),#857,.F.);
#6643=ADVANCED_FACE('',(#992),#6574,.F.);
#6644=ADVANCED_FACE('',(#993,#786),#858,.F.);
#6645=ADVANCED_FACE('',(#994),#6575,.F.);
#6646=ADVANCED_FACE('',(#995),#6576,.F.);
#6647=ADVANCED_FACE('',(#996,#787),#859,.F.);
#6648=ADVANCED_FACE('',(#997),#6577,.F.);
#6649=ADVANCED_FACE('',(#998,#788),#860,.F.);
#6650=ADVANCED_FACE('',(#999),#6578,.F.);
#6651=ADVANCED_FACE('',(#1000,#789),#861,.F.);
#6652=ADVANCED_FACE('',(#1001),#6579,.F.);
#6653=ADVANCED_FACE('',(#1002),#759,.F.);
#6654=ADVANCED_FACE('',(#1003),#6580,.T.);
#6655=ADVANCED_FACE('',(#1004,#790),#862,.T.);
#6656=ADVANCED_FACE('',(#1005),#667,.T.);
#6657=ADVANCED_FACE('',(#1006,#791),#863,.T.);
#6658=ADVANCED_FACE('',(#1007),#864,.T.);
#6659=ADVANCED_FACE('',(#1008),#668,.T.);
#6660=ADVANCED_FACE('',(#1009),#865,.T.);
#6661=ADVANCED_FACE('',(#1010),#669,.T.);
#6662=ADVANCED_FACE('',(#1011),#866,.T.);
#6663=ADVANCED_FACE('',(#1012),#670,.T.);
#6664=ADVANCED_FACE('',(#1013),#867,.T.);
#6665=ADVANCED_FACE('',(#1014),#671,.T.);
#6666=ADVANCED_FACE('',(#1015),#6581,.T.);
#6667=ADVANCED_FACE('',(#1016,#792),#868,.T.);
#6668=ADVANCED_FACE('',(#1017),#6582,.T.);
#6669=ADVANCED_FACE('',(#1018),#869,.F.);
#6670=ADVANCED_FACE('',(#1019),#672,.T.);
#6671=ADVANCED_FACE('',(#1020),#870,.T.);
#6672=ADVANCED_FACE('',(#1021),#673,.T.);
#6673=ADVANCED_FACE('',(#1022),#871,.T.);
#6674=ADVANCED_FACE('',(#1023),#674,.T.);
#6675=ADVANCED_FACE('',(#1024),#872,.T.);
#6676=ADVANCED_FACE('',(#1025),#675,.T.);
#6677=ADVANCED_FACE('',(#1026),#873,.T.);
#6678=ADVANCED_FACE('',(#1027,#793),#874,.T.);
#6679=ADVANCED_FACE('',(#1028),#676,.F.);
#6680=ADVANCED_FACE('',(#1029),#875,.T.);
#6681=ADVANCED_FACE('',(#1030),#677,.F.);
#6682=ADVANCED_FACE('',(#1031),#876,.T.);
#6683=ADVANCED_FACE('',(#1032),#678,.F.);
#6684=ADVANCED_FACE('',(#1033),#877,.T.);
#6685=ADVANCED_FACE('',(#1034),#679,.F.);
#6686=ADVANCED_FACE('',(#1035),#878,.T.);
#6687=ADVANCED_FACE('',(#1036,#794),#879,.F.);
#6688=ADVANCED_FACE('',(#1037),#6583,.F.);
#6689=ADVANCED_FACE('',(#1038),#880,.F.);
#6690=ADVANCED_FACE('',(#1039),#6584,.F.);
#6691=ADVANCED_FACE('',(#1040,#795),#881,.F.);
#6692=ADVANCED_FACE('',(#1041,#796),#882,.F.);
#6693=ADVANCED_FACE('',(#1042),#6585,.F.);
#6694=ADVANCED_FACE('',(#1043),#6586,.F.);
#6695=ADVANCED_FACE('',(#1044),#883,.T.);
#6696=ADVANCED_FACE('',(#1045),#6587,.T.);
#6697=ADVANCED_FACE('',(#1046,#797),#884,.T.);
#6698=ADVANCED_FACE('',(#1047),#6588,.T.);
#6699=ADVANCED_FACE('',(#1048),#885,.T.);
#7025=CLOSED_SHELL('',(#6630,#6631,#6632,#6633,#6634,#6635,#6636,#6637,
#6638,#6639,#6640,#6641,#6642,#6643,#6644,#6645,#6646,#6647,#6648,#6649,
#6650,#6651,#6652,#6653,#6654,#6655,#6656,#6657,#6658,#6659,#6660,#6661,
#6662,#6663,#6664,#6665,#6666,#6667,#6668,#6669,#6670,#6671,#6672,#6673,
#6674,#6675,#6676,#6677,#6678,#6679,#6680,#6681,#6682,#6683,#6684,#6685,
#6686,#6687,#6688,#6689,#6690,#6691,#6692,#6693,#6694,#6695,#6696,#6697,
#6698,#6699));
#7147=AXIS2_PLACEMENT_3D('',#9461,#7833,#7834);
#7148=AXIS2_PLACEMENT_3D('',#9462,#7835,#7836);
#7149=AXIS2_PLACEMENT_3D('',#9464,#7837,#7838);
#7150=AXIS2_PLACEMENT_3D('',#9467,#7840,#7841);
#7151=AXIS2_PLACEMENT_3D('',#9468,#7842,#7843);
#7152=AXIS2_PLACEMENT_3D('',#9470,#7844,#7845);
#7153=AXIS2_PLACEMENT_3D('',#9471,#7846,#7847);
#7154=AXIS2_PLACEMENT_3D('',#9474,#7849,#7850);
#7155=AXIS2_PLACEMENT_3D('',#9475,#7851,#7852);
#7156=AXIS2_PLACEMENT_3D('',#9477,#7853,#7854);
#7157=AXIS2_PLACEMENT_3D('',#9478,#7855,#7856);
#7158=AXIS2_PLACEMENT_3D('',#9481,#7858,#7859);
#7159=AXIS2_PLACEMENT_3D('',#9482,#7860,#7861);
#7160=AXIS2_PLACEMENT_3D('',#9484,#7862,#7863);
#7161=AXIS2_PLACEMENT_3D('',#9485,#7864,#7865);
#7162=AXIS2_PLACEMENT_3D('',#9488,#7867,#7868);
#7163=AXIS2_PLACEMENT_3D('',#9489,#7869,#7870);
#7164=AXIS2_PLACEMENT_3D('',#9491,#7871,#7872);
#7165=AXIS2_PLACEMENT_3D('',#9492,#7873,#7874);
#7166=AXIS2_PLACEMENT_3D('',#9495,#7876,#7877);
#7167=AXIS2_PLACEMENT_3D('',#9496,#7878,#7879);
#7168=AXIS2_PLACEMENT_3D('',#9498,#7880,#7881);
#7169=AXIS2_PLACEMENT_3D('',#9501,#7883,#7884);
#7170=AXIS2_PLACEMENT_3D('',#9502,#7885,#7886);
#7171=AXIS2_PLACEMENT_3D('',#9504,#7887,#7888);
#7172=AXIS2_PLACEMENT_3D('',#9505,#7889,#7890);
#7173=AXIS2_PLACEMENT_3D('',#9508,#7892,#7893);
#7174=AXIS2_PLACEMENT_3D('',#9509,#7894,#7895);
#7175=AXIS2_PLACEMENT_3D('',#9511,#7896,#7897);
#7176=AXIS2_PLACEMENT_3D('',#9512,#7898,#7899);
#7177=AXIS2_PLACEMENT_3D('',#9515,#7901,#7902);
#7178=AXIS2_PLACEMENT_3D('',#9516,#7903,#7904);
#7179=AXIS2_PLACEMENT_3D('',#9518,#7905,#7906);
#7180=AXIS2_PLACEMENT_3D('',#9519,#7907,#7908);
#7181=AXIS2_PLACEMENT_3D('',#9522,#7910,#7911);
#7182=AXIS2_PLACEMENT_3D('',#9523,#7912,#7913);
#7183=AXIS2_PLACEMENT_3D('',#9525,#7914,#7915);
#7184=AXIS2_PLACEMENT_3D('',#9528,#7917,#7918);
#7185=AXIS2_PLACEMENT_3D('',#9529,#7919,#7920);
#7186=AXIS2_PLACEMENT_3D('',#9531,#7921,#7922);
#7187=AXIS2_PLACEMENT_3D('',#9532,#7923,#7924);
#7188=AXIS2_PLACEMENT_3D('',#9535,#7926,#7927);
#7189=AXIS2_PLACEMENT_3D('',#9536,#7928,#7929);
#7190=AXIS2_PLACEMENT_3D('',#9538,#7930,#7931);
#7191=AXIS2_PLACEMENT_3D('',#9539,#7932,#7933);
#7192=AXIS2_PLACEMENT_3D('',#9542,#7935,#7936);
#7193=AXIS2_PLACEMENT_3D('',#9543,#7937,#7938);
#7194=AXIS2_PLACEMENT_3D('',#9545,#7939,#7940);
#7195=AXIS2_PLACEMENT_3D('',#9546,#7941,#7942);
#7196=AXIS2_PLACEMENT_3D('',#9549,#7944,#7945);
#7197=AXIS2_PLACEMENT_3D('',#9550,#7946,#7947);
#7198=AXIS2_PLACEMENT_3D('',#9553,#7948,#7949);
#7199=AXIS2_PLACEMENT_3D('',#9555,#7950,#7951);
#7200=AXIS2_PLACEMENT_3D('',#9556,#7952,#7953);
#7201=AXIS2_PLACEMENT_3D('',#9557,#7954,#7955);
#7202=AXIS2_PLACEMENT_3D('',#9558,#7956,#7957);
#7203=AXIS2_PLACEMENT_3D('',#9562,#7959,#7960);
#7204=AXIS2_PLACEMENT_3D('',#9563,#7961,#7962);
#7205=AXIS2_PLACEMENT_3D('',#9564,#7963,#7964);
#7206=AXIS2_PLACEMENT_3D('',#9569,#7966,#7967);
#7207=AXIS2_PLACEMENT_3D('',#9573,#7969,#7970);
#7208=AXIS2_PLACEMENT_3D('',#9577,#7972,#7973);
#7209=AXIS2_PLACEMENT_3D('',#9580,#7975,#7976);
#7210=AXIS2_PLACEMENT_3D('',#9581,#7977,#7978);
#7211=AXIS2_PLACEMENT_3D('',#9584,#7980,#7981);
#7212=AXIS2_PLACEMENT_3D('',#9585,#7982,#7983);
#7213=AXIS2_PLACEMENT_3D('',#9586,#7984,#7985);
#7214=AXIS2_PLACEMENT_3D('',#9592,#7989,#7990);
#7215=AXIS2_PLACEMENT_3D('',#9594,#7991,#7992);
#7216=AXIS2_PLACEMENT_3D('',#9596,#7994,#7995);
#7217=AXIS2_PLACEMENT_3D('',#9600,#7998,#7999);
#7218=AXIS2_PLACEMENT_3D('',#9602,#8000,#8001);
#7219=AXIS2_PLACEMENT_3D('',#9604,#8003,#8004);
#7220=AXIS2_PLACEMENT_3D('',#9608,#8007,#8008);
#7221=AXIS2_PLACEMENT_3D('',#9610,#8009,#8010);
#7222=AXIS2_PLACEMENT_3D('',#9612,#8012,#8013);
#7223=AXIS2_PLACEMENT_3D('',#9616,#8016,#8017);
#7224=AXIS2_PLACEMENT_3D('',#9617,#8018,#8019);
#7225=AXIS2_PLACEMENT_3D('',#9618,#8020,#8021);
#7226=AXIS2_PLACEMENT_3D('',#9622,#8023,#8024);
#7227=AXIS2_PLACEMENT_3D('',#9624,#8026,#8027);
#7228=AXIS2_PLACEMENT_3D('',#9628,#8030,#8031);
#7229=AXIS2_PLACEMENT_3D('',#9631,#8033,#8034);
#7230=AXIS2_PLACEMENT_3D('',#9632,#8035,#8036);
#7231=AXIS2_PLACEMENT_3D('',#9636,#8039,#8040);
#7232=AXIS2_PLACEMENT_3D('',#9641,#8043,#8044);
#7233=AXIS2_PLACEMENT_3D('',#9642,#8045,#8046);
#7234=AXIS2_PLACEMENT_3D('',#9648,#8050,#8051);
#7235=AXIS2_PLACEMENT_3D('',#9652,#8053,#8054);
#7236=AXIS2_PLACEMENT_3D('',#9653,#8055,#8056);
#7237=AXIS2_PLACEMENT_3D('',#9654,#8057,#8058);
#7238=AXIS2_PLACEMENT_3D('',#9660,#8062,#8063);
#7239=AXIS2_PLACEMENT_3D('',#9663,#8065,#8066);
#7240=AXIS2_PLACEMENT_3D('',#9664,#8067,#8068);
#7241=AXIS2_PLACEMENT_3D('',#9665,#8069,#8070);
#7242=AXIS2_PLACEMENT_3D('',#9669,#8073,#8074);
#7243=AXIS2_PLACEMENT_3D('',#9672,#8076,#8077);
#7244=AXIS2_PLACEMENT_3D('',#9673,#8078,#8079);
#7245=AXIS2_PLACEMENT_3D('',#9675,#8081,#8082);
#7246=AXIS2_PLACEMENT_3D('',#9678,#8083,#8084);
#7247=AXIS2_PLACEMENT_3D('',#9682,#8086,#8087);
#7248=AXIS2_PLACEMENT_3D('',#9686,#8089,#8090);
#7249=AXIS2_PLACEMENT_3D('',#9690,#8092,#8093);
#7250=AXIS2_PLACEMENT_3D('',#9692,#8095,#8096);
#7251=AXIS2_PLACEMENT_3D('',#9696,#8098,#8099);
#7252=AXIS2_PLACEMENT_3D('',#9698,#8101,#8102);
#7253=AXIS2_PLACEMENT_3D('',#9702,#8105,#8106);
#7254=AXIS2_PLACEMENT_3D('',#9705,#8108,#8109);
#7255=AXIS2_PLACEMENT_3D('',#9706,#8110,#8111);
#7256=AXIS2_PLACEMENT_3D('',#9710,#8114,#8115);
#7257=AXIS2_PLACEMENT_3D('',#9713,#8117,#8118);
#7258=AXIS2_PLACEMENT_3D('',#9714,#8119,#8120);
#7259=AXIS2_PLACEMENT_3D('',#9718,#8123,#8124);
#7260=AXIS2_PLACEMENT_3D('',#9721,#8126,#8127);
#7261=AXIS2_PLACEMENT_3D('',#9722,#8128,#8129);
#7262=AXIS2_PLACEMENT_3D('',#9724,#8131,#8132);
#7263=AXIS2_PLACEMENT_3D('',#9730,#8136,#8137);
#7264=AXIS2_PLACEMENT_3D('',#9733,#8139,#8140);
#7265=AXIS2_PLACEMENT_3D('',#9734,#8141,#8142);
#7266=AXIS2_PLACEMENT_3D('',#9738,#8145,#8146);
#7267=AXIS2_PLACEMENT_3D('',#9741,#8148,#8149);
#7268=AXIS2_PLACEMENT_3D('',#9742,#8150,#8151);
#7269=AXIS2_PLACEMENT_3D('',#9746,#8153,#8154);
#7270=AXIS2_PLACEMENT_3D('',#9749,#8156,#8157);
#7271=AXIS2_PLACEMENT_3D('',#9750,#8158,#8159);
#7272=AXIS2_PLACEMENT_3D('',#9752,#8161,#8162);
#7273=AXIS2_PLACEMENT_3D('',#9754,#8164,#8165);
#7274=AXIS2_PLACEMENT_3D('',#9756,#8167,#8168);
#7275=AXIS2_PLACEMENT_3D('',#9757,#8169,#8170);
#7276=AXIS2_PLACEMENT_3D('',#9760,#8173,#8174);
#7277=AXIS2_PLACEMENT_3D('',#9762,#8176,#8177);
#7278=AXIS2_PLACEMENT_3D('',#9763,#8178,#8179);
#7833=DIRECTION('axis',(0.,0.,1.));
#7834=DIRECTION('refdir',(1.,0.,0.));
#7835=DIRECTION('center_axis',(0.,-1.,0.));
#7836=DIRECTION('ref_axis',(1.,0.,0.));
#7837=DIRECTION('center_axis',(0.,-1.,0.));
#7838=DIRECTION('ref_axis',(1.,0.,0.));
#7839=DIRECTION('',(0.,-1.,0.));
#7840=DIRECTION('center_axis',(0.,-1.,0.));
#7841=DIRECTION('ref_axis',(1.,0.,0.));
#7842=DIRECTION('center_axis',(0.,1.,0.));
#7843=DIRECTION('ref_axis',(0.,0.,1.));
#7844=DIRECTION('center_axis',(0.,-1.,0.));
#7845=DIRECTION('ref_axis',(1.,0.,0.));
#7846=DIRECTION('center_axis',(0.,-1.,0.));
#7847=DIRECTION('ref_axis',(1.,0.,0.));
#7848=DIRECTION('',(0.,-1.,0.));
#7849=DIRECTION('center_axis',(0.,-1.,0.));
#7850=DIRECTION('ref_axis',(1.,0.,0.));
#7851=DIRECTION('center_axis',(0.,-1.,0.));
#7852=DIRECTION('ref_axis',(0.,0.,-1.));
#7853=DIRECTION('center_axis',(0.,-1.,0.));
#7854=DIRECTION('ref_axis',(1.,0.,0.));
#7855=DIRECTION('center_axis',(0.,-1.,0.));
#7856=DIRECTION('ref_axis',(1.,0.,0.));
#7857=DIRECTION('',(0.,-1.,0.));
#7858=DIRECTION('center_axis',(0.,-1.,0.));
#7859=DIRECTION('ref_axis',(1.,0.,0.));
#7860=DIRECTION('center_axis',(0.,-1.,0.));
#7861=DIRECTION('ref_axis',(0.,0.,-1.));
#7862=DIRECTION('center_axis',(0.,-1.,0.));
#7863=DIRECTION('ref_axis',(1.,0.,0.));
#7864=DIRECTION('center_axis',(0.,-1.,0.));
#7865=DIRECTION('ref_axis',(1.,0.,0.));
#7866=DIRECTION('',(0.,-1.,0.));
#7867=DIRECTION('center_axis',(0.,-1.,0.));
#7868=DIRECTION('ref_axis',(1.,0.,0.));
#7869=DIRECTION('center_axis',(0.,1.,0.));
#7870=DIRECTION('ref_axis',(0.,0.,1.));
#7871=DIRECTION('center_axis',(0.,-1.,0.));
#7872=DIRECTION('ref_axis',(1.,0.,0.));
#7873=DIRECTION('center_axis',(0.,-1.,0.));
#7874=DIRECTION('ref_axis',(1.,0.,0.));
#7875=DIRECTION('',(0.,-1.,0.));
#7876=DIRECTION('center_axis',(0.,1.,0.));
#7877=DIRECTION('ref_axis',(1.,0.,0.));
#7878=DIRECTION('center_axis',(1.,0.,0.));
#7879=DIRECTION('ref_axis',(0.,1.,0.));
#7880=DIRECTION('center_axis',(1.,0.,0.));
#7881=DIRECTION('ref_axis',(0.,1.,0.));
#7882=DIRECTION('',(1.,0.,0.));
#7883=DIRECTION('center_axis',(1.,0.,0.));
#7884=DIRECTION('ref_axis',(0.,0.,-1.));
#7885=DIRECTION('center_axis',(-1.,0.,0.));
#7886=DIRECTION('ref_axis',(0.,0.,1.));
#7887=DIRECTION('center_axis',(1.,0.,0.));
#7888=DIRECTION('ref_axis',(0.,0.,-1.));
#7889=DIRECTION('center_axis',(1.,0.,0.));
#7890=DIRECTION('ref_axis',(0.,1.,0.));
#7891=DIRECTION('',(1.,0.,0.));
#7892=DIRECTION('center_axis',(1.,0.,0.));
#7893=DIRECTION('ref_axis',(0.,0.,-1.));
#7894=DIRECTION('center_axis',(1.,0.,0.));
#7895=DIRECTION('ref_axis',(0.,0.,-1.));
#7896=DIRECTION('center_axis',(1.,0.,0.));
#7897=DIRECTION('ref_axis',(0.,0.,-1.));
#7898=DIRECTION('center_axis',(1.,0.,0.));
#7899=DIRECTION('ref_axis',(0.,1.,0.));
#7900=DIRECTION('',(1.,0.,0.));
#7901=DIRECTION('center_axis',(1.,0.,0.));
#7902=DIRECTION('ref_axis',(0.,0.,-1.));
#7903=DIRECTION('center_axis',(1.,0.,0.));
#7904=DIRECTION('ref_axis',(0.,0.,-1.));
#7905=DIRECTION('center_axis',(1.,0.,0.));
#7906=DIRECTION('ref_axis',(0.,0.,-1.));
#7907=DIRECTION('center_axis',(1.,0.,0.));
#7908=DIRECTION('ref_axis',(0.,1.,0.));
#7909=DIRECTION('',(1.,0.,0.));
#7910=DIRECTION('center_axis',(-1.,0.,0.));
#7911=DIRECTION('ref_axis',(0.,1.,0.));
#7912=DIRECTION('center_axis',(1.,0.,0.));
#7913=DIRECTION('ref_axis',(0.,1.,0.));
#7914=DIRECTION('center_axis',(1.,0.,0.));
#7915=DIRECTION('ref_axis',(0.,1.,0.));
#7916=DIRECTION('',(1.,0.,0.));
#7917=DIRECTION('center_axis',(1.,0.,0.));
#7918=DIRECTION('ref_axis',(0.,0.,-1.));
#7919=DIRECTION('center_axis',(-1.,0.,0.));
#7920=DIRECTION('ref_axis',(0.,0.,1.));
#7921=DIRECTION('center_axis',(1.,0.,0.));
#7922=DIRECTION('ref_axis',(0.,0.,-1.));
#7923=DIRECTION('center_axis',(1.,0.,0.));
#7924=DIRECTION('ref_axis',(0.,1.,0.));
#7925=DIRECTION('',(1.,0.,0.));
#7926=DIRECTION('center_axis',(1.,0.,0.));
#7927=DIRECTION('ref_axis',(0.,0.,-1.));
#7928=DIRECTION('center_axis',(-1.,0.,0.));
#7929=DIRECTION('ref_axis',(0.,0.,1.));
#7930=DIRECTION('center_axis',(1.,0.,0.));
#7931=DIRECTION('ref_axis',(0.,0.,-1.));
#7932=DIRECTION('center_axis',(1.,0.,0.));
#7933=DIRECTION('ref_axis',(0.,1.,0.));
#7934=DIRECTION('',(1.,0.,0.));
#7935=DIRECTION('center_axis',(1.,0.,0.));
#7936=DIRECTION('ref_axis',(0.,0.,-1.));
#7937=DIRECTION('center_axis',(1.,0.,0.));
#7938=DIRECTION('ref_axis',(0.,0.,-1.));
#7939=DIRECTION('center_axis',(1.,0.,0.));
#7940=DIRECTION('ref_axis',(0.,0.,-1.));
#7941=DIRECTION('center_axis',(1.,0.,0.));
#7942=DIRECTION('ref_axis',(0.,1.,0.));
#7943=DIRECTION('',(1.,0.,0.));
#7944=DIRECTION('center_axis',(-1.,0.,0.));
#7945=DIRECTION('ref_axis',(0.,1.,0.));
#7946=DIRECTION('center_axis',(0.,-1.,0.));
#7947=DIRECTION('ref_axis',(0.,0.,-1.));
#7948=DIRECTION('center_axis',(0.,-1.,0.));
#7949=DIRECTION('ref_axis',(1.,0.,0.));
#7950=DIRECTION('center_axis',(-1.,0.,-1.22464679914735E-16));
#7951=DIRECTION('ref_axis',(-1.22464679914735E-16,0.,1.));
#7952=DIRECTION('center_axis',(0.,1.,0.));
#7953=DIRECTION('ref_axis',(1.,0.,0.));
#7954=DIRECTION('center_axis',(0.,-1.,0.));
#7955=DIRECTION('ref_axis',(1.,0.,0.));
#7956=DIRECTION('center_axis',(0.,-1.,0.));
#7957=DIRECTION('ref_axis',(1.,0.,0.));
#7958=DIRECTION('',(0.,1.,0.));
#7959=DIRECTION('center_axis',(0.,1.,0.));
#7960=DIRECTION('ref_axis',(-1.,0.,0.));
#7961=DIRECTION('center_axis',(0.,1.,0.));
#7962=DIRECTION('ref_axis',(-1.,0.,0.));
#7963=DIRECTION('center_axis',(0.,1.,0.));
#7964=DIRECTION('ref_axis',(-1.,0.,0.));
#7965=DIRECTION('',(1.,0.,0.));
#7966=DIRECTION('center_axis',(0.,-1.,0.));
#7967=DIRECTION('ref_axis',(-0.707106781186548,0.,-0.707106781186547));
#7968=DIRECTION('',(0.,0.,-1.));
#7969=DIRECTION('center_axis',(0.,-1.,0.));
#7970=DIRECTION('ref_axis',(-0.707106781186549,0.,0.707106781186546));
#7971=DIRECTION('',(-1.,0.,0.));
#7972=DIRECTION('center_axis',(0.,-1.,0.));
#7973=DIRECTION('ref_axis',(0.707106781186549,0.,0.707106781186546));
#7974=DIRECTION('',(0.,0.,1.));
#7975=DIRECTION('center_axis',(0.,-1.,0.));
#7976=DIRECTION('ref_axis',(0.707106781186548,0.,-0.707106781186547));
#7977=DIRECTION('center_axis',(0.,-1.,0.));
#7978=DIRECTION('ref_axis',(-1.,0.,0.));
#7979=DIRECTION('',(-0.707106781186549,0.707106781186546,-8.65956056235495E-17));
#7980=DIRECTION('center_axis',(0.,-1.,0.));
#7981=DIRECTION('ref_axis',(-1.,0.,0.));
#7982=DIRECTION('center_axis',(0.,1.,0.));
#7983=DIRECTION('ref_axis',(0.,0.,1.));
#7984=DIRECTION('center_axis',(0.,0.707106781186548,-0.707106781186548));
#7985=DIRECTION('ref_axis',(-1.,0.,0.));
#7986=DIRECTION('',(0.,0.707106781186548,0.707106781186548));
#7987=DIRECTION('',(0.,-0.707106781186548,-0.707106781186548));
#7988=DIRECTION('',(-1.,0.,0.));
#7989=DIRECTION('center_axis',(0.,-1.,0.));
#7990=DIRECTION('ref_axis',(-0.707106781186548,0.,-0.707106781186547));
#7991=DIRECTION('center_axis',(0.,1.,0.));
#7992=DIRECTION('ref_axis',(-0.707106781186548,0.,-0.707106781186547));
#7993=DIRECTION('',(0.707106781186545,0.70710678118655,0.));
#7994=DIRECTION('center_axis',(-0.707106781186548,0.707106781186548,0.));
#7995=DIRECTION('ref_axis',(0.,0.,1.));
#7996=DIRECTION('',(0.707106781186548,0.707106781186548,0.));
#7997=DIRECTION('',(0.,0.,1.));
#7998=DIRECTION('center_axis',(0.,-1.,0.));
#7999=DIRECTION('ref_axis',(-0.707106781186549,0.,0.707106781186546));
#8000=DIRECTION('center_axis',(0.,1.,0.));
#8001=DIRECTION('ref_axis',(-0.707106781186549,0.,0.707106781186546));
#8002=DIRECTION('',(0.,0.707106781186555,-0.70710678118654));
#8003=DIRECTION('center_axis',(0.,0.707106781186548,0.707106781186548));
#8004=DIRECTION('ref_axis',(1.,0.,0.));
#8005=DIRECTION('',(1.,0.,0.));
#8006=DIRECTION('',(0.,0.707106781186548,-0.707106781186548));
#8007=DIRECTION('center_axis',(0.,-1.,0.));
#8008=DIRECTION('ref_axis',(0.707106781186549,0.,0.707106781186546));
#8009=DIRECTION('center_axis',(0.,1.,0.));
#8010=DIRECTION('ref_axis',(0.707106781186549,0.,0.707106781186546));
#8011=DIRECTION('',(-0.707106781186549,0.707106781186546,0.));
#8012=DIRECTION('center_axis',(0.707106781186548,0.707106781186548,0.));
#8013=DIRECTION('ref_axis',(0.,0.,-1.));
#8014=DIRECTION('',(0.,0.,-1.));
#8015=DIRECTION('',(-0.707106781186548,0.707106781186548,0.));
#8016=DIRECTION('center_axis',(0.,-1.,0.));
#8017=DIRECTION('ref_axis',(0.707106781186548,0.,-0.707106781186547));
#8018=DIRECTION('center_axis',(0.,1.,0.));
#8019=DIRECTION('ref_axis',(0.707106781186548,0.,-0.707106781186547));
#8020=DIRECTION('center_axis',(0.,-1.,0.));
#8021=DIRECTION('ref_axis',(-0.707106781186549,0.,0.707106781186546));
#8022=DIRECTION('',(0.,-1.,0.));
#8023=DIRECTION('center_axis',(0.,-1.,0.));
#8024=DIRECTION('ref_axis',(-0.707106781186549,0.,0.707106781186546));
#8025=DIRECTION('',(0.,1.,0.));
#8026=DIRECTION('center_axis',(-1.,0.,0.));
#8027=DIRECTION('ref_axis',(0.,-1.,0.));
#8028=DIRECTION('',(0.,1.,0.));
#8029=DIRECTION('',(0.,0.,-1.));
#8030=DIRECTION('center_axis',(0.,-1.,0.));
#8031=DIRECTION('ref_axis',(-0.707106781186548,0.,-0.707106781186547));
#8032=DIRECTION('',(0.,-1.,0.));
#8033=DIRECTION('center_axis',(0.,-1.,0.));
#8034=DIRECTION('ref_axis',(-0.707106781186548,0.,-0.707106781186547));
#8035=DIRECTION('center_axis',(0.,0.,1.));
#8036=DIRECTION('ref_axis',(1.,0.,0.));
#8037=DIRECTION('',(0.,1.,0.));
#8038=DIRECTION('',(1.,0.,0.));
#8039=DIRECTION('center_axis',(0.,1.,0.));
#8040=DIRECTION('ref_axis',(-0.707106781186549,0.,0.707106781186546));
#8041=DIRECTION('',(0.,0.707106781186554,0.707106781186541));
#8042=DIRECTION('',(0.707106781186549,-0.707106781186546,0.));
#8043=DIRECTION('center_axis',(0.,1.,0.));
#8044=DIRECTION('ref_axis',(-0.707106781186549,0.,0.707106781186546));
#8045=DIRECTION('center_axis',(0.,-0.707106781186546,0.707106781186549));
#8046=DIRECTION('ref_axis',(1.,0.,0.));
#8047=DIRECTION('',(0.,0.707106781186549,0.707106781186546));
#8048=DIRECTION('',(-1.,0.,0.));
#8049=DIRECTION('',(1.,0.,0.));
#8050=DIRECTION('center_axis',(0.,1.,0.));
#8051=DIRECTION('ref_axis',(0.707106781186549,0.,0.707106781186546));
#8052=DIRECTION('',(0.707106781186547,0.707106781186547,0.));
#8053=DIRECTION('center_axis',(0.,-1.,0.));
#8054=DIRECTION('ref_axis',(0.707106781186549,0.,0.707106781186546));
#8055=DIRECTION('center_axis',(0.,1.,0.));
#8056=DIRECTION('ref_axis',(0.707106781186549,0.,0.707106781186546));
#8057=DIRECTION('center_axis',(0.707106781186549,-0.707106781186546,0.));
#8058=DIRECTION('ref_axis',(0.,0.,-1.));
#8059=DIRECTION('',(0.,0.,-1.));
#8060=DIRECTION('',(0.707106781186546,0.707106781186549,0.));
#8061=DIRECTION('',(0.,0.,1.));
#8062=DIRECTION('center_axis',(0.,1.,0.));
#8063=DIRECTION('ref_axis',(0.707106781186548,0.,-0.707106781186547));
#8064=DIRECTION('',(0.,0.707106781186549,-0.707106781186546));
#8065=DIRECTION('center_axis',(0.,-1.,0.));
#8066=DIRECTION('ref_axis',(0.707106781186548,0.,-0.707106781186547));
#8067=DIRECTION('center_axis',(0.,1.,0.));
#8068=DIRECTION('ref_axis',(0.707106781186548,0.,-0.707106781186547));
#8069=DIRECTION('center_axis',(0.,-0.707106781186548,-0.707106781186548));
#8070=DIRECTION('ref_axis',(-1.,0.,0.));
#8071=DIRECTION('',(-1.,0.,0.));
#8072=DIRECTION('',(0.,0.707106781186546,-0.707106781186549));
#8073=DIRECTION('center_axis',(0.,1.,0.));
#8074=DIRECTION('ref_axis',(-0.707106781186548,0.,-0.707106781186547));
#8075=DIRECTION('',(-0.707106781186549,0.707106781186546,0.));
#8076=DIRECTION('center_axis',(0.,1.,0.));
#8077=DIRECTION('ref_axis',(-0.707106781186548,0.,-0.707106781186547));
#8078=DIRECTION('center_axis',(-0.707106781186548,-0.707106781186547,0.));
#8079=DIRECTION('ref_axis',(0.,0.,1.));
#8080=DIRECTION('',(0.,0.,1.));
#8081=DIRECTION('center_axis',(0.,-1.,0.));
#8082=DIRECTION('ref_axis',(1.,0.,0.));
#8083=DIRECTION('center_axis',(0.,-1.,0.));
#8084=DIRECTION('ref_axis',(-0.707106781186546,0.,0.707106781186549));
#8085=DIRECTION('',(-1.,0.,0.));
#8086=DIRECTION('center_axis',(0.,-1.,0.));
#8087=DIRECTION('ref_axis',(0.707106781186546,0.,0.707106781186549));
#8088=DIRECTION('',(0.,0.,1.));
#8089=DIRECTION('center_axis',(0.,-1.,0.));
#8090=DIRECTION('ref_axis',(0.707106781186548,0.,-0.707106781186548));
#8091=DIRECTION('',(1.,0.,0.));
#8092=DIRECTION('center_axis',(0.,-1.,0.));
#8093=DIRECTION('ref_axis',(-0.707106781186548,0.,-0.707106781186548));
#8094=DIRECTION('',(0.,0.,-1.));
#8095=DIRECTION('center_axis',(0.,-1.,0.));
#8096=DIRECTION('ref_axis',(-0.707106781186546,0.,0.707106781186549));
#8097=DIRECTION('',(0.707106781186547,0.707106781186547,6.28036983473509E-15));
#8098=DIRECTION('center_axis',(0.,1.,0.));
#8099=DIRECTION('ref_axis',(-0.707106781186546,0.,0.707106781186549));
#8100=DIRECTION('',(0.,-0.707106781186549,0.707106781186546));
#8101=DIRECTION('center_axis',(0.707106781186548,-0.707106781186547,0.));
#8102=DIRECTION('ref_axis',(0.,0.,-1.));
#8103=DIRECTION('',(0.707106781186547,0.707106781186547,0.));
#8104=DIRECTION('',(0.,0.,1.));
#8105=DIRECTION('center_axis',(0.,-1.,0.));
#8106=DIRECTION('ref_axis',(-0.707106781186548,0.,-0.707106781186548));
#8107=DIRECTION('',(0.,0.707106781186549,0.707106781186546));
#8108=DIRECTION('center_axis',(0.,1.,0.));
#8109=DIRECTION('ref_axis',(-0.707106781186547,0.,-0.707106781186547));
#8110=DIRECTION('center_axis',(0.,-0.707106781186548,0.707106781186548));
#8111=DIRECTION('ref_axis',(1.,0.,0.));
#8112=DIRECTION('',(0.,0.707106781186547,0.707106781186547));
#8113=DIRECTION('',(-1.,0.,0.));
#8114=DIRECTION('center_axis',(0.,-1.,0.));
#8115=DIRECTION('ref_axis',(0.707106781186548,0.,-0.707106781186548));
#8116=DIRECTION('',(-0.707106781186546,0.707106781186549,0.));
#8117=DIRECTION('center_axis',(0.,1.,0.));
#8118=DIRECTION('ref_axis',(0.707106781186547,0.,-0.707106781186547));
#8119=DIRECTION('center_axis',(-0.707106781186546,-0.707106781186549,0.));
#8120=DIRECTION('ref_axis',(0.,0.,1.));
#8121=DIRECTION('',(-0.707106781186549,0.707106781186546,0.));
#8122=DIRECTION('',(0.,0.,-1.));
#8123=DIRECTION('center_axis',(0.,-1.,0.));
#8124=DIRECTION('ref_axis',(0.707106781186546,0.,0.707106781186549));
#8125=DIRECTION('',(0.,0.707106781186549,-0.707106781186546));
#8126=DIRECTION('center_axis',(0.,1.,0.));
#8127=DIRECTION('ref_axis',(0.707106781186546,0.,0.707106781186549));
#8128=DIRECTION('center_axis',(0.,-0.707106781186546,-0.707106781186549));
#8129=DIRECTION('ref_axis',(-1.,0.,0.));
#8130=DIRECTION('',(1.,0.,0.));
#8131=DIRECTION('center_axis',(1.,0.,0.));
#8132=DIRECTION('ref_axis',(0.,1.,0.));
#8133=DIRECTION('',(0.,-1.,0.));
#8134=DIRECTION('',(0.,0.,1.));
#8135=DIRECTION('',(0.,1.,0.));
#8136=DIRECTION('center_axis',(0.,1.,0.));
#8137=DIRECTION('ref_axis',(0.707106781186546,0.,0.707106781186549));
#8138=DIRECTION('',(0.,1.,0.));
#8139=DIRECTION('center_axis',(0.,-1.,0.));
#8140=DIRECTION('ref_axis',(0.707106781186546,0.,0.707106781186549));
#8141=DIRECTION('center_axis',(0.,0.,1.));
#8142=DIRECTION('ref_axis',(1.,0.,0.));
#8143=DIRECTION('',(0.,-1.,0.));
#8144=DIRECTION('',(-1.,0.,0.));
#8145=DIRECTION('center_axis',(0.,-1.,0.));
#8146=DIRECTION('ref_axis',(-0.707106781186546,0.,0.707106781186549));
#8147=DIRECTION('',(0.,1.,0.));
#8148=DIRECTION('center_axis',(0.,-1.,0.));
#8149=DIRECTION('ref_axis',(-0.707106781186546,0.,0.707106781186549));
#8150=DIRECTION('center_axis',(0.,1.,0.));
#8151=DIRECTION('ref_axis',(-1.,0.,0.));
#8152=DIRECTION('',(0.,0.,1.));
#8153=DIRECTION('center_axis',(0.,-1.,0.));
#8154=DIRECTION('ref_axis',(-0.707106781186547,0.,-0.707106781186547));
#8155=DIRECTION('',(-1.,0.,0.));
#8156=DIRECTION('center_axis',(0.,-1.,0.));
#8157=DIRECTION('ref_axis',(0.707106781186547,0.,-0.707106781186547));
#8158=DIRECTION('center_axis',(-1.,0.,0.));
#8159=DIRECTION('ref_axis',(0.,-1.,0.));
#8160=DIRECTION('',(0.,-1.,0.));
#8161=DIRECTION('center_axis',(0.,-1.,0.));
#8162=DIRECTION('ref_axis',(-0.707106781186547,0.,-0.707106781186547));
#8163=DIRECTION('',(0.,1.,0.));
#8164=DIRECTION('center_axis',(0.,1.,0.));
#8165=DIRECTION('ref_axis',(0.707106781186547,0.,-0.707106781186547));
#8166=DIRECTION('',(0.,-1.,0.));
#8167=DIRECTION('center_axis',(0.,0.,1.));
#8168=DIRECTION('ref_axis',(1.,0.,0.));
#8169=DIRECTION('center_axis',(0.,1.,0.));
#8170=DIRECTION('ref_axis',(0.707106781186549,0.,0.707106781186546));
#8171=DIRECTION('',(0.,-1.,0.));
#8172=DIRECTION('',(0.,1.,0.));
#8173=DIRECTION('center_axis',(1.,0.,0.));
#8174=DIRECTION('ref_axis',(0.,1.,0.));
#8175=DIRECTION('',(0.,-1.,0.));
#8176=DIRECTION('center_axis',(0.,1.,0.));
#8177=DIRECTION('ref_axis',(0.707106781186548,0.,-0.707106781186547));
#8178=DIRECTION('center_axis',(0.,0.,1.));
#8179=DIRECTION('ref_axis',(1.,0.,0.));
#9461=CARTESIAN_POINT('',(0.,0.,0.));
#9462=CARTESIAN_POINT('Origin',(0.,54.15,55.));
#9463=CARTESIAN_POINT('',(-14.,54.,55.));
#9464=CARTESIAN_POINT('Origin',(0.,54.,55.));
#9465=CARTESIAN_POINT('',(-14.,53.3,55.));
#9466=CARTESIAN_POINT('',(-14.,54.15,55.));
#9467=CARTESIAN_POINT('Origin',(0.,53.3,55.));
#9468=CARTESIAN_POINT('Origin',(14.7,53.3,55.));
#9469=CARTESIAN_POINT('',(-14.7,53.3,55.));
#9470=CARTESIAN_POINT('Origin',(0.,53.3,55.));
#9471=CARTESIAN_POINT('Origin',(0.,52.65,55.));
#9472=CARTESIAN_POINT('',(-14.7,52.,55.));
#9473=CARTESIAN_POINT('',(-14.7,52.65,55.));
#9474=CARTESIAN_POINT('Origin',(0.,52.,55.));
#9475=CARTESIAN_POINT('Origin',(14.,52.,55.));
#9476=CARTESIAN_POINT('',(-14.,52.,55.));
#9477=CARTESIAN_POINT('Origin',(0.,52.,55.));
#9478=CARTESIAN_POINT('Origin',(0.,48.,55.));
#9479=CARTESIAN_POINT('',(-14.,44.,55.));
#9480=CARTESIAN_POINT('',(-14.,48.,55.));
#9481=CARTESIAN_POINT('Origin',(0.,44.,55.));
#9482=CARTESIAN_POINT('Origin',(12.,44.,55.));
#9483=CARTESIAN_POINT('',(-12.,44.,55.));
#9484=CARTESIAN_POINT('Origin',(0.,44.,55.));
#9485=CARTESIAN_POINT('Origin',(0.,41.,55.));
#9486=CARTESIAN_POINT('',(-12.,38.,55.));
#9487=CARTESIAN_POINT('',(-12.,41.,55.));
#9488=CARTESIAN_POINT('Origin',(0.,38.,55.));
#9489=CARTESIAN_POINT('Origin',(14.,38.,55.));
#9490=CARTESIAN_POINT('',(-14.,38.,55.));
#9491=CARTESIAN_POINT('Origin',(0.,38.,55.));
#9492=CARTESIAN_POINT('Origin',(0.,32.5,55.));
#9493=CARTESIAN_POINT('',(-14.,28.,55.));
#9494=CARTESIAN_POINT('',(-14.,32.5,55.));
#9495=CARTESIAN_POINT('Origin',(0.,28.,55.));
#9496=CARTESIAN_POINT('Origin',(-40.15,0.,55.));
#9497=CARTESIAN_POINT('',(-40.,-14.,55.));
#9498=CARTESIAN_POINT('Origin',(-40.,0.,55.));
#9499=CARTESIAN_POINT('',(-39.3,-14.,55.));
#9500=CARTESIAN_POINT('',(-40.15,-14.,55.));
#9501=CARTESIAN_POINT('Origin',(-39.3,0.,55.));
#9502=CARTESIAN_POINT('Origin',(-39.3,14.7,55.));
#9503=CARTESIAN_POINT('',(-39.3,-14.7,55.));
#9504=CARTESIAN_POINT('Origin',(-39.3,0.,55.));
#9505=CARTESIAN_POINT('Origin',(-38.65,0.,55.));
#9506=CARTESIAN_POINT('',(-38.,-14.7,55.));
#9507=CARTESIAN_POINT('',(-38.65,-14.7,55.));
#9508=CARTESIAN_POINT('Origin',(-38.,0.,55.));
#9509=CARTESIAN_POINT('Origin',(-38.,14.,55.));
#9510=CARTESIAN_POINT('',(-38.,-14.,55.));
#9511=CARTESIAN_POINT('Origin',(-38.,0.,55.));
#9512=CARTESIAN_POINT('Origin',(-34.,0.,55.));
#9513=CARTESIAN_POINT('',(-30.,-14.,55.));
#9514=CARTESIAN_POINT('',(-34.,-14.,55.));
#9515=CARTESIAN_POINT('Origin',(-30.,0.,55.));
#9516=CARTESIAN_POINT('Origin',(-30.,12.,55.));
#9517=CARTESIAN_POINT('',(-30.,-12.,55.));
#9518=CARTESIAN_POINT('Origin',(-30.,0.,55.));
#9519=CARTESIAN_POINT('Origin',(-28.5,0.,55.));
#9520=CARTESIAN_POINT('',(-28.,-12.,55.));
#9521=CARTESIAN_POINT('',(-28.5,-12.,55.));
#9522=CARTESIAN_POINT('Origin',(-28.,0.,55.));
#9523=CARTESIAN_POINT('Origin',(28.5,0.,55.));
#9524=CARTESIAN_POINT('',(28.,-12.,55.));
#9525=CARTESIAN_POINT('Origin',(28.,0.,55.));
#9526=CARTESIAN_POINT('',(30.,-12.,55.));
#9527=CARTESIAN_POINT('',(28.5,-12.,55.));
#9528=CARTESIAN_POINT('Origin',(30.,0.,55.));
#9529=CARTESIAN_POINT('Origin',(30.,14.,55.));
#9530=CARTESIAN_POINT('',(30.,-14.,55.));
#9531=CARTESIAN_POINT('Origin',(30.,0.,55.));
#9532=CARTESIAN_POINT('Origin',(34.,0.,55.));
#9533=CARTESIAN_POINT('',(38.,-14.,55.));
#9534=CARTESIAN_POINT('',(34.,-14.,55.));
#9535=CARTESIAN_POINT('Origin',(38.,0.,55.));
#9536=CARTESIAN_POINT('Origin',(38.,14.7,55.));
#9537=CARTESIAN_POINT('',(38.,-14.7,55.));
#9538=CARTESIAN_POINT('Origin',(38.,0.,55.));
#9539=CARTESIAN_POINT('Origin',(38.65,0.,55.));
#9540=CARTESIAN_POINT('',(39.3,-14.7,55.));
#9541=CARTESIAN_POINT('',(38.65,-14.7,55.));
#9542=CARTESIAN_POINT('Origin',(39.3,0.,55.));
#9543=CARTESIAN_POINT('Origin',(39.3,14.,55.));
#9544=CARTESIAN_POINT('',(39.3,-14.,55.));
#9545=CARTESIAN_POINT('Origin',(39.3,0.,55.));
#9546=CARTESIAN_POINT('Origin',(40.15,0.,55.));
#9547=CARTESIAN_POINT('',(40.,-14.,55.));
#9548=CARTESIAN_POINT('',(40.15,-14.,55.));
#9549=CARTESIAN_POINT('Origin',(40.,0.,55.));
#9550=CARTESIAN_POINT('Origin',(0.,41.5,55.));
#9551=CARTESIAN_POINT('',(-20.,41.5,55.));
#9552=CARTESIAN_POINT('',(-2.44929359829471E-15,41.5,75.));
#9553=CARTESIAN_POINT('Origin',(0.,41.5,55.));
#9554=CARTESIAN_POINT('',(-2.63299061816681E-15,40.,76.5));
#9555=CARTESIAN_POINT('Origin',(-2.63299061816681E-15,41.5,76.5));
#9556=CARTESIAN_POINT('Origin',(0.,40.,55.));
#9557=CARTESIAN_POINT('Origin',(0.,41.5,55.));
#9558=CARTESIAN_POINT('Origin',(0.,46.75,55.));
#9559=CARTESIAN_POINT('',(-20.,53.,55.));
#9560=CARTESIAN_POINT('',(-20.,46.75,55.));
#9561=CARTESIAN_POINT('',(20.,53.,55.));
#9562=CARTESIAN_POINT('Origin',(0.,53.,55.));
#9563=CARTESIAN_POINT('Origin',(0.,53.,55.));
#9564=CARTESIAN_POINT('Origin',(40.,40.,15.));
#9565=CARTESIAN_POINT('',(-38.,40.,15.8));
#9566=CARTESIAN_POINT('',(38.,40.,15.8));
#9567=CARTESIAN_POINT('',(20.,40.,15.8));
#9568=CARTESIAN_POINT('',(-39.2,40.,17.));
#9569=CARTESIAN_POINT('Origin',(-38.,40.,17.));
#9570=CARTESIAN_POINT('',(-39.2,40.,93.));
#9571=CARTESIAN_POINT('',(-39.2,40.,15.));
#9572=CARTESIAN_POINT('',(-38.,40.,94.2));
#9573=CARTESIAN_POINT('Origin',(-38.,40.,93.));
#9574=CARTESIAN_POINT('',(38.,40.,94.2));
#9575=CARTESIAN_POINT('',(20.,40.,94.2));
#9576=CARTESIAN_POINT('',(39.2,40.,93.));
#9577=CARTESIAN_POINT('Origin',(38.,40.,93.));
#9578=CARTESIAN_POINT('',(39.2,40.,17.));
#9579=CARTESIAN_POINT('',(39.2,40.,15.));
#9580=CARTESIAN_POINT('Origin',(38.,40.,17.));
#9581=CARTESIAN_POINT('Origin',(0.,53.5,55.));
#9582=CARTESIAN_POINT('',(19.,54.,55.));
#9583=CARTESIAN_POINT('',(19.5,53.5,55.));
#9584=CARTESIAN_POINT('Origin',(0.,54.,55.));
#9585=CARTESIAN_POINT('Origin',(20.,54.,55.));
#9586=CARTESIAN_POINT('Origin',(20.,39.6,15.4));
#9587=CARTESIAN_POINT('',(-38.,39.2,15.));
#9588=CARTESIAN_POINT('',(-38.,39.2,15.));
#9589=CARTESIAN_POINT('',(38.,39.2,15.));
#9590=CARTESIAN_POINT('',(38.,40.,15.8));
#9591=CARTESIAN_POINT('',(20.,39.2,15.));
#9592=CARTESIAN_POINT('Origin',(-38.,39.6,17.));
#9593=CARTESIAN_POINT('',(-40.,39.2,17.));
#9594=CARTESIAN_POINT('Origin',(-38.,39.2,17.));
#9595=CARTESIAN_POINT('',(-40.,39.2,17.));
#9596=CARTESIAN_POINT('Origin',(-39.6,39.6,15.));
#9597=CARTESIAN_POINT('',(-40.,39.2,93.));
#9598=CARTESIAN_POINT('',(-40.,39.2,93.));
#9599=CARTESIAN_POINT('',(-40.,39.2,15.));
#9600=CARTESIAN_POINT('Origin',(-38.,39.6,93.));
#9601=CARTESIAN_POINT('',(-38.,39.2,95.));
#9602=CARTESIAN_POINT('Origin',(-38.,39.2,93.));
#9603=CARTESIAN_POINT('',(-38.,39.2,95.));
#9604=CARTESIAN_POINT('Origin',(20.,39.6,94.6));
#9605=CARTESIAN_POINT('',(38.,39.2,95.));
#9606=CARTESIAN_POINT('',(20.,39.2,95.));
#9607=CARTESIAN_POINT('',(38.,39.2,95.));
#9608=CARTESIAN_POINT('Origin',(38.,39.6,93.));
#9609=CARTESIAN_POINT('',(40.,39.2,93.));
#9610=CARTESIAN_POINT('Origin',(38.,39.2,93.));
#9611=CARTESIAN_POINT('',(40.,39.2,93.));
#9612=CARTESIAN_POINT('Origin',(39.6,39.6,15.));
#9613=CARTESIAN_POINT('',(40.,39.2,17.));
#9614=CARTESIAN_POINT('',(40.,39.2,15.));
#9615=CARTESIAN_POINT('',(40.,39.2,17.));
#9616=CARTESIAN_POINT('Origin',(38.,39.6,17.));
#9617=CARTESIAN_POINT('Origin',(38.,39.2,17.));
#9618=CARTESIAN_POINT('Origin',(-38.,25.,93.));
#9619=CARTESIAN_POINT('',(-40.,-19.,93.));
#9620=CARTESIAN_POINT('',(-40.,25.,93.));
#9621=CARTESIAN_POINT('',(-38.,-19.,95.));
#9622=CARTESIAN_POINT('Origin',(-38.,-19.,93.));
#9623=CARTESIAN_POINT('',(-38.,25.,95.));
#9624=CARTESIAN_POINT('Origin',(-40.,40.,15.));
#9625=CARTESIAN_POINT('',(-40.,-19.,17.));
#9626=CARTESIAN_POINT('',(-40.,25.,17.));
#9627=CARTESIAN_POINT('',(-40.,-19.,15.));
#9628=CARTESIAN_POINT('Origin',(-38.,25.,17.));
#9629=CARTESIAN_POINT('',(-38.,-19.,15.));
#9630=CARTESIAN_POINT('',(-38.,25.,15.));
#9631=CARTESIAN_POINT('Origin',(-38.,-19.,17.));
#9632=CARTESIAN_POINT('Origin',(0.,10.,15.));
#9633=CARTESIAN_POINT('',(38.,-19.,15.));
#9634=CARTESIAN_POINT('',(38.,-5.,15.));
#9635=CARTESIAN_POINT('',(-20.,-19.,15.));
#9636=CARTESIAN_POINT('Origin',(-38.,-19.5,93.));
#9637=CARTESIAN_POINT('',(-38.,-20.,94.));
#9638=CARTESIAN_POINT('',(-38.,-20.,94.));
#9639=CARTESIAN_POINT('',(-39.,-20.,93.));
#9640=CARTESIAN_POINT('',(-40.,-19.,93.));
#9641=CARTESIAN_POINT('Origin',(-38.,-20.,93.));
#9642=CARTESIAN_POINT('Origin',(-20.,-19.5,94.5));
#9643=CARTESIAN_POINT('',(38.,-20.,94.));
#9644=CARTESIAN_POINT('',(38.,-19.,95.));
#9645=CARTESIAN_POINT('',(38.,-20.,94.));
#9646=CARTESIAN_POINT('',(-20.,-19.,95.));
#9647=CARTESIAN_POINT('',(-20.,-20.,94.));
#9648=CARTESIAN_POINT('Origin',(38.,-19.5,93.));
#9649=CARTESIAN_POINT('',(39.,-20.,93.));
#9650=CARTESIAN_POINT('',(40.,-19.,93.));
#9651=CARTESIAN_POINT('',(39.,-20.,93.));
#9652=CARTESIAN_POINT('Origin',(38.,-19.,93.));
#9653=CARTESIAN_POINT('Origin',(38.,-20.,93.));
#9654=CARTESIAN_POINT('Origin',(39.5,-19.5,15.));
#9655=CARTESIAN_POINT('',(39.,-20.,17.));
#9656=CARTESIAN_POINT('',(39.,-20.,15.));
#9657=CARTESIAN_POINT('',(40.,-19.,17.));
#9658=CARTESIAN_POINT('',(39.,-20.,17.));
#9659=CARTESIAN_POINT('',(40.,-19.,15.));
#9660=CARTESIAN_POINT('Origin',(38.,-19.5,17.));
#9661=CARTESIAN_POINT('',(38.,-20.,16.));
#9662=CARTESIAN_POINT('',(38.,-20.,16.));
#9663=CARTESIAN_POINT('Origin',(38.,-19.,17.));
#9664=CARTESIAN_POINT('Origin',(38.,-20.,17.));
#9665=CARTESIAN_POINT('Origin',(-20.,-19.5,15.5));
#9666=CARTESIAN_POINT('',(-38.,-20.,16.));
#9667=CARTESIAN_POINT('',(-20.,-20.,16.));
#9668=CARTESIAN_POINT('',(-38.,-20.,16.));
#9669=CARTESIAN_POINT('Origin',(-38.,-19.5,17.));
#9670=CARTESIAN_POINT('',(-39.,-20.,17.));
#9671=CARTESIAN_POINT('',(-39.,-20.,17.));
#9672=CARTESIAN_POINT('Origin',(-38.,-20.,17.));
#9673=CARTESIAN_POINT('Origin',(-39.5,-19.5,15.));
#9674=CARTESIAN_POINT('',(-39.,-20.,15.));
#9675=CARTESIAN_POINT('Origin',(-40.,-20.,15.));
#9676=CARTESIAN_POINT('',(-25.,-20.,84.));
#9677=CARTESIAN_POINT('',(-29.,-20.,80.));
#9678=CARTESIAN_POINT('Origin',(-25.,-20.,80.));
#9679=CARTESIAN_POINT('',(25.,-20.,84.));
#9680=CARTESIAN_POINT('',(-20.,-20.,84.));
#9681=CARTESIAN_POINT('',(29.,-20.,80.));
#9682=CARTESIAN_POINT('Origin',(25.,-20.,80.));
#9683=CARTESIAN_POINT('',(29.,-20.,30.));
#9684=CARTESIAN_POINT('',(29.,-20.,21.));
#9685=CARTESIAN_POINT('',(25.,-20.,26.));
#9686=CARTESIAN_POINT('Origin',(25.,-20.,30.));
#9687=CARTESIAN_POINT('',(-25.,-20.,26.));
#9688=CARTESIAN_POINT('',(-20.,-20.,26.));
#9689=CARTESIAN_POINT('',(-29.,-20.,30.));
#9690=CARTESIAN_POINT('Origin',(-25.,-20.,30.));
#9691=CARTESIAN_POINT('',(-29.,-20.,21.));
#9692=CARTESIAN_POINT('Origin',(-25.,-19.5,80.));
#9693=CARTESIAN_POINT('',(-28.,-19.,80.));
#9694=CARTESIAN_POINT('',(-29.,-20.,80.));
#9695=CARTESIAN_POINT('',(-25.,-19.,83.));
#9696=CARTESIAN_POINT('Origin',(-25.,-19.,80.));
#9697=CARTESIAN_POINT('',(-25.,-19.,83.));
#9698=CARTESIAN_POINT('Origin',(-28.5,-19.5,21.));
#9699=CARTESIAN_POINT('',(-28.,-19.,30.));
#9700=CARTESIAN_POINT('',(-29.,-20.,30.));
#9701=CARTESIAN_POINT('',(-28.,-19.,21.));
#9702=CARTESIAN_POINT('Origin',(-25.,-19.5,30.));
#9703=CARTESIAN_POINT('',(-25.,-19.,27.));
#9704=CARTESIAN_POINT('',(-25.,-20.,26.));
#9705=CARTESIAN_POINT('Origin',(-25.,-19.,30.));
#9706=CARTESIAN_POINT('Origin',(-20.,-19.5,26.5));
#9707=CARTESIAN_POINT('',(25.,-19.,27.));
#9708=CARTESIAN_POINT('',(25.,-20.,26.));
#9709=CARTESIAN_POINT('',(-20.,-19.,27.));
#9710=CARTESIAN_POINT('Origin',(25.,-19.5,30.));
#9711=CARTESIAN_POINT('',(28.,-19.,30.));
#9712=CARTESIAN_POINT('',(29.,-20.,30.));
#9713=CARTESIAN_POINT('Origin',(25.,-19.,30.));
#9714=CARTESIAN_POINT('Origin',(28.5,-19.5,21.));
#9715=CARTESIAN_POINT('',(28.,-19.,80.));
#9716=CARTESIAN_POINT('',(29.,-20.,80.));
#9717=CARTESIAN_POINT('',(28.,-19.,21.));
#9718=CARTESIAN_POINT('Origin',(25.,-19.5,80.));
#9719=CARTESIAN_POINT('',(25.,-19.,83.));
#9720=CARTESIAN_POINT('',(25.,-20.,84.));
#9721=CARTESIAN_POINT('Origin',(25.,-19.,80.));
#9722=CARTESIAN_POINT('Origin',(-20.,-19.5,83.5));
#9723=CARTESIAN_POINT('',(-20.,-19.,83.));
#9724=CARTESIAN_POINT('Origin',(28.,-21.,27.));
#9725=CARTESIAN_POINT('',(28.,28.,80.));
#9726=CARTESIAN_POINT('',(28.,-8.75,80.));
#9727=CARTESIAN_POINT('',(28.,28.,30.));
#9728=CARTESIAN_POINT('',(28.,28.,27.));
#9729=CARTESIAN_POINT('',(28.,-8.75,30.));
#9730=CARTESIAN_POINT('Origin',(25.,-8.75,80.));
#9731=CARTESIAN_POINT('',(25.,28.,83.));
#9732=CARTESIAN_POINT('',(25.,-8.75,83.));
#9733=CARTESIAN_POINT('Origin',(25.,28.,80.));
#9734=CARTESIAN_POINT('Origin',(0.,3.5,83.));
#9735=CARTESIAN_POINT('',(-25.,28.,83.));
#9736=CARTESIAN_POINT('',(-25.,15.75,83.));
#9737=CARTESIAN_POINT('',(28.,28.,83.));
#9738=CARTESIAN_POINT('Origin',(-25.,15.75,80.));
#9739=CARTESIAN_POINT('',(-28.,28.,80.));
#9740=CARTESIAN_POINT('',(-28.,15.75,80.));
#9741=CARTESIAN_POINT('Origin',(-25.,28.,80.));
#9742=CARTESIAN_POINT('Origin',(28.,28.,27.));
#9743=CARTESIAN_POINT('',(-28.,28.,30.));
#9744=CARTESIAN_POINT('',(-28.,28.,27.));
#9745=CARTESIAN_POINT('',(-25.,28.,27.));
#9746=CARTESIAN_POINT('Origin',(-25.,28.,30.));
#9747=CARTESIAN_POINT('',(25.,28.,27.));
#9748=CARTESIAN_POINT('',(28.,28.,27.));
#9749=CARTESIAN_POINT('Origin',(25.,28.,30.));
#9750=CARTESIAN_POINT('Origin',(-28.,28.,27.));
#9751=CARTESIAN_POINT('',(-28.,15.75,30.));
#9752=CARTESIAN_POINT('Origin',(-25.,15.75,30.));
#9753=CARTESIAN_POINT('',(-25.,15.75,27.));
#9754=CARTESIAN_POINT('Origin',(25.,-8.75,30.));
#9755=CARTESIAN_POINT('',(25.,-8.75,27.));
#9756=CARTESIAN_POINT('Origin',(0.,3.5,27.));
#9757=CARTESIAN_POINT('Origin',(38.,-5.,93.));
#9758=CARTESIAN_POINT('',(38.,-5.,95.));
#9759=CARTESIAN_POINT('',(40.,-5.,93.));
#9760=CARTESIAN_POINT('Origin',(40.,-20.,15.));
#9761=CARTESIAN_POINT('',(40.,-5.,17.));
#9762=CARTESIAN_POINT('Origin',(38.,-5.,17.));
#9763=CARTESIAN_POINT('Origin',(0.,10.,95.));
#23232=UNCERTAINTY_MEASURE_WITH_UNIT(LENGTH_MEASURE(0.01),#23255,
'DISTANCE_ACCURACY_VALUE',
'Maximum model space distance between geometric entities at asserted c
onnectivities');
#23242=UNCERTAINTY_MEASURE_WITH_UNIT(LENGTH_MEASURE(0.01),#23255,
'DISTANCE_ACCURACY_VALUE',
'Maximum model space distance between geometric entities at asserted c
onnectivities');
#23244=(
GEOMETRIC_REPRESENTATION_CONTEXT(3)
GLOBAL_UNCERTAINTY_ASSIGNED_CONTEXT((#23232))
GLOBAL_UNIT_ASSIGNED_CONTEXT((#23255,#23257,#23258))
REPRESENTATION_CONTEXT('','3D')
);
#23254=(
GEOMETRIC_REPRESENTATION_CONTEXT(3)
GLOBAL_UNCERTAINTY_ASSIGNED_CONTEXT((#23242))
GLOBAL_UNIT_ASSIGNED_CONTEXT((#23255,#23257,#23258))
REPRESENTATION_CONTEXT('','3D')
);
#23255=(
LENGTH_UNIT()
NAMED_UNIT(*)
SI_UNIT(.MILLI.,.METRE.)
);
#23257=(
NAMED_UNIT(*)
PLANE_ANGLE_UNIT()
SI_UNIT($,.RADIAN.)
);
#23258=(
NAMED_UNIT(*)
SI_UNIT($,.STERADIAN.)
SOLID_ANGLE_UNIT()
);
#23260=SHAPE_DEFINITION_REPRESENTATION(#23271,#23300);
#23271=PRODUCT_DEFINITION_SHAPE('',$,#23312);
#23300=SHAPE_REPRESENTATION('',(#7147),#23244);
#23310=PRODUCT_DEFINITION_CONTEXT('part definition',#23345,'design');
#23312=PRODUCT_DEFINITION('2026-10-11-09-11-47-549',
'01_Aluminium_Gearbox_Block_Front_Window',#23323,#23310);
#23323=PRODUCT_DEFINITION_FORMATION('',$,#23348);
#23345=APPLICATION_CONTEXT(
'Core Data for Automotive Mechanical Design Process');
#23346=PRODUCT_CONTEXT('part definition',#23345,'mechanical');
#23348=PRODUCT('2026-10-11-09-11-47-549',
'01_Aluminium_Gearbox_Block_Front_Window',$,(#23346));
#23435=COLOUR_RGB('Dark Blue',0.08,0.2,0.34);
#23436=FILL_AREA_STYLE_COLOUR('',#23435);
#23437=FILL_AREA_STYLE('',(#23436));
#23438=SURFACE_STYLE_FILL_AREA(#23437);
#23439=SURFACE_SIDE_STYLE('',(#23438));
#23440=SURFACE_STYLE_USAGE(.BOTH.,#23439);
#23441=PRESENTATION_STYLE_ASSIGNMENT((#23440));
ENDSEC;
END-ISO-10303-21;
